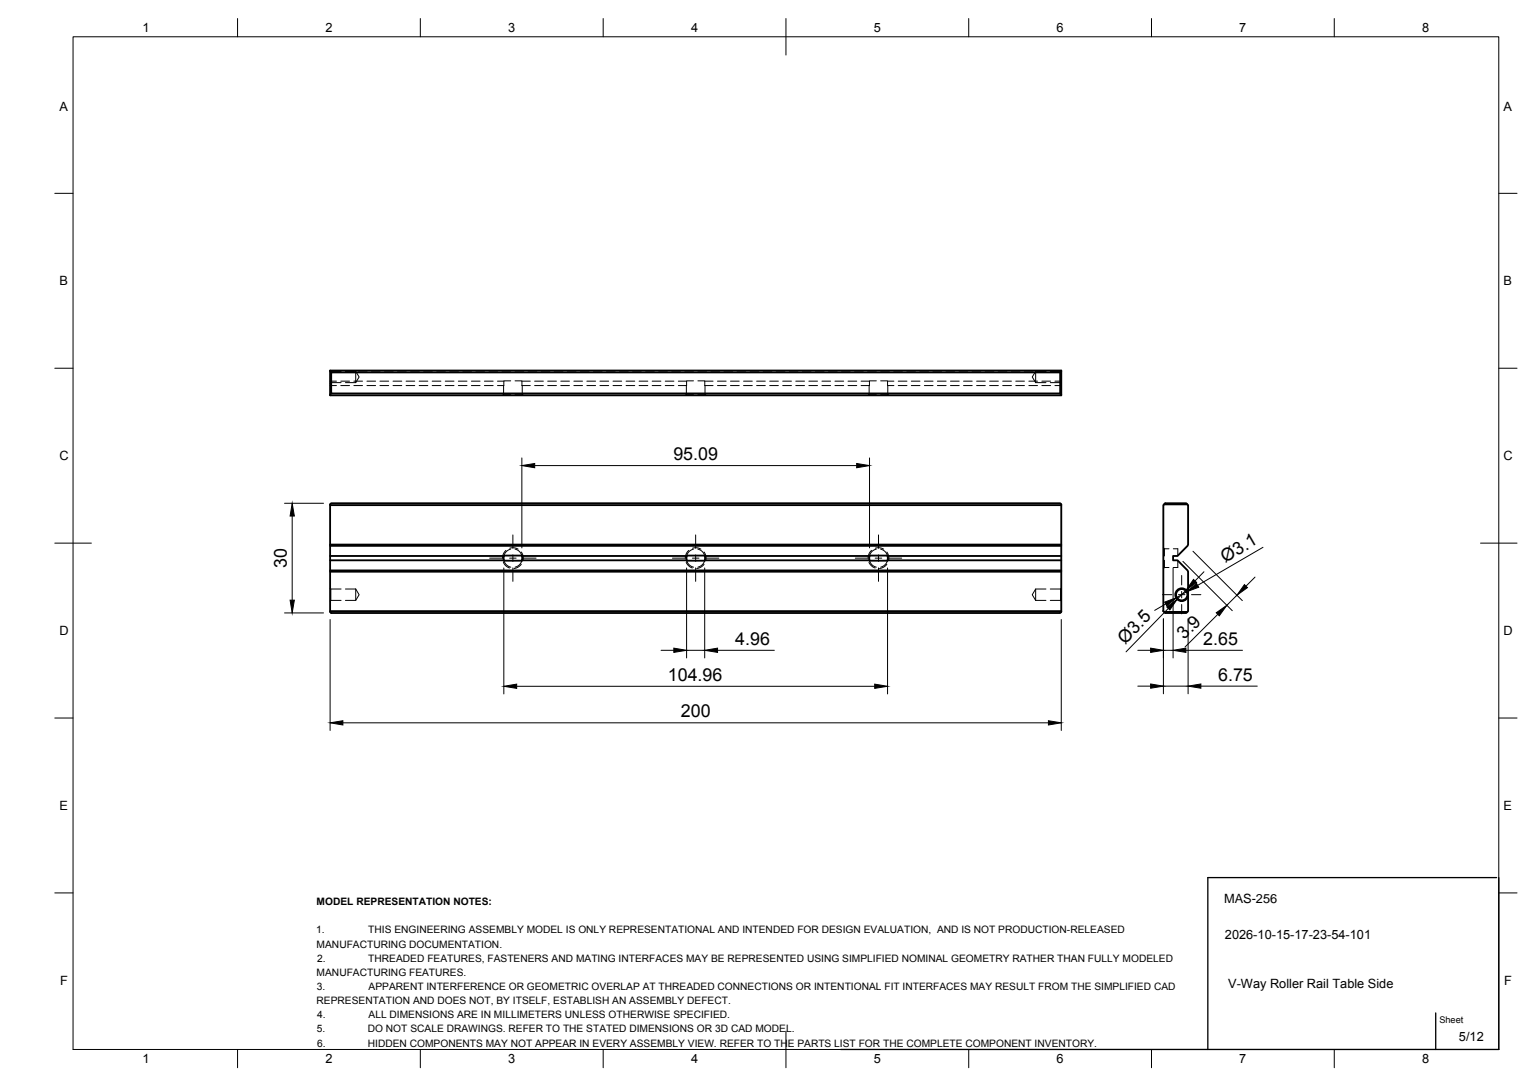
ISO-10303-21;
HEADER;
/* Generated by software containing ST-Developer
 * from STEP Tools, Inc. (www.steptools.com) 
 */

FILE_DESCRIPTION(
/* description */ (''),
/* implementation_level */ '2;1');

FILE_NAME(
/* name */ 'V-Way Roller Rail Table Side.step',
/* time_stamp */ '2026-10-14T18:40:07-07:00',
/* author */ (''),
/* organization */ (''),
/* preprocessor_version */ 'ST-DEVELOPER v20.2',
/* originating_system */ 'Autodesk Translation Framework v15.15.0.0',
/* authorisation */ '');

FILE_SCHEMA (('AUTOMOTIVE_DESIGN { 1 0 10303 214 3 1 1 }'));
ENDSEC;

DATA;
#10=MECHANICAL_DESIGN_GEOMETRIC_PRESENTATION_REPRESENTATION('',(#833),#81040);
#372=ELLIPSE('',#15639,3.6062445840514,2.55000000000001);
#373=ELLIPSE('',#15641,3.6062445840514,2.55000000000001);
#374=ELLIPSE('',#15643,3.6062445840514,2.55000000000001);
#375=ELLIPSE('',#15645,3.6062445840514,2.55000000000001);
#376=ELLIPSE('',#15651,3.6062445840514,2.55000000000001);
#377=ELLIPSE('',#15653,3.6062445840514,2.55000000000001);
#378=ELLIPSE('',#15655,3.6062445840514,2.55000000000001);
#379=ELLIPSE('',#15657,3.6062445840514,2.55000000000001);
#380=ELLIPSE('',#15663,3.60624458405139,2.55);
#381=ELLIPSE('',#15665,3.60624458405139,2.55);
#382=ELLIPSE('',#15667,3.60624458405139,2.55);
#383=ELLIPSE('',#15669,3.60624458405139,2.55);
#813=SHAPE_REPRESENTATION_RELATIONSHIP('SRR','None',#81132,#823);
#823=ADVANCED_BREP_SHAPE_REPRESENTATION('',(#843),#81032);
#833=STYLED_ITEM('',(#81191),#843);
#843=MANIFOLD_SOLID_BREP('Body1',#15086);
#915=CYLINDRICAL_SURFACE('',#15619,1.55);
#916=CYLINDRICAL_SURFACE('',#15627,1.55);
#917=CYLINDRICAL_SURFACE('',#15637,2.55000000000001);
#918=CYLINDRICAL_SURFACE('',#15649,2.55000000000001);
#919=CYLINDRICAL_SURFACE('',#15661,2.55);
#1169=FACE_BOUND('',#2653,.T.);
#1170=FACE_BOUND('',#2654,.T.);
#1171=FACE_BOUND('',#2655,.T.);
#1283=PLANE('',#15618);
#1284=PLANE('',#15626);
#1285=PLANE('',#15634);
#1286=PLANE('',#15671);
#1287=PLANE('',#15672);
#1288=PLANE('',#15673);
#1289=PLANE('',#15674);
#1290=PLANE('',#15675);
#1291=PLANE('',#15676);
#1292=PLANE('',#15677);
#1293=PLANE('',#15678);
#1294=PLANE('',#15679);
#1295=PLANE('',#15680);
#1296=PLANE('',#15681);
#1297=PLANE('',#15682);
#1298=PLANE('',#15683);
#1299=PLANE('',#15684);
#1300=PLANE('',#15685);
#1301=PLANE('',#15686);
#1302=PLANE('',#15687);
#1303=PLANE('',#15688);
#1304=PLANE('',#15689);
#1305=PLANE('',#15690);
#1306=PLANE('',#15691);
#1307=PLANE('',#15692);
#1308=PLANE('',#15693);
#1309=PLANE('',#15694);
#1310=PLANE('',#15695);
#1311=PLANE('',#15696);
#1312=PLANE('',#15697);
#1313=PLANE('',#15698);
#1314=PLANE('',#15699);
#1315=PLANE('',#15700);
#1316=PLANE('',#15701);
#1317=PLANE('',#15702);
#1318=PLANE('',#15703);
#1319=PLANE('',#15704);
#1814=FACE_OUTER_BOUND('',#2643,.T.);
#1815=FACE_OUTER_BOUND('',#2644,.T.);
#1816=FACE_OUTER_BOUND('',#2645,.T.);
#1817=FACE_OUTER_BOUND('',#2646,.T.);
#1818=FACE_OUTER_BOUND('',#2647,.T.);
#1819=FACE_OUTER_BOUND('',#2648,.T.);
#1820=FACE_OUTER_BOUND('',#2649,.T.);
#1821=FACE_OUTER_BOUND('',#2650,.T.);
#1822=FACE_OUTER_BOUND('',#2651,.T.);
#1823=FACE_OUTER_BOUND('',#2652,.T.);
#1824=FACE_OUTER_BOUND('',#2656,.T.);
#1825=FACE_OUTER_BOUND('',#2657,.T.);
#1826=FACE_OUTER_BOUND('',#2658,.T.);
#1827=FACE_OUTER_BOUND('',#2659,.T.);
#1828=FACE_OUTER_BOUND('',#2660,.T.);
#1829=FACE_OUTER_BOUND('',#2661,.T.);
#1830=FACE_OUTER_BOUND('',#2662,.T.);
#1831=FACE_OUTER_BOUND('',#2663,.T.);
#1832=FACE_OUTER_BOUND('',#2664,.T.);
#1833=FACE_OUTER_BOUND('',#2665,.T.);
#1834=FACE_OUTER_BOUND('',#2666,.T.);
#1835=FACE_OUTER_BOUND('',#2667,.T.);
#1836=FACE_OUTER_BOUND('',#2668,.T.);
#1837=FACE_OUTER_BOUND('',#2669,.T.);
#1838=FACE_OUTER_BOUND('',#2670,.T.);
#1839=FACE_OUTER_BOUND('',#2671,.T.);
#1840=FACE_OUTER_BOUND('',#2672,.T.);
#1841=FACE_OUTER_BOUND('',#2673,.T.);
#1842=FACE_OUTER_BOUND('',#2674,.T.);
#1843=FACE_OUTER_BOUND('',#2675,.T.);
#1844=FACE_OUTER_BOUND('',#2676,.T.);
#1845=FACE_OUTER_BOUND('',#2677,.T.);
#1846=FACE_OUTER_BOUND('',#2678,.T.);
#1847=FACE_OUTER_BOUND('',#2679,.T.);
#1848=FACE_OUTER_BOUND('',#2680,.T.);
#1849=FACE_OUTER_BOUND('',#2681,.T.);
#1850=FACE_OUTER_BOUND('',#2682,.T.);
#1851=FACE_OUTER_BOUND('',#2683,.T.);
#1852=FACE_OUTER_BOUND('',#2684,.T.);
#1853=FACE_OUTER_BOUND('',#2685,.T.);
#1854=FACE_OUTER_BOUND('',#2686,.T.);
#1855=FACE_OUTER_BOUND('',#2687,.T.);
#1856=FACE_OUTER_BOUND('',#2688,.T.);
#1857=FACE_OUTER_BOUND('',#2689,.T.);
#1858=FACE_OUTER_BOUND('',#2690,.T.);
#1859=FACE_OUTER_BOUND('',#2691,.T.);
#1860=FACE_OUTER_BOUND('',#2692,.T.);
#1861=FACE_OUTER_BOUND('',#2693,.T.);
#1862=FACE_OUTER_BOUND('',#2694,.T.);
#2643=EDGE_LOOP('',(#10770,#10771,#10772,#10773));
#2644=EDGE_LOOP('',(#10774,#10775,#10776,#10777,#10778,#10779,#10780,#10781,
#10782,#10783,#10784,#10785,#10786,#10787,#10788,#10789,#10790,#10791));
#2645=EDGE_LOOP('',(#10792,#10793,#10794,#10795,#10796));
#2646=EDGE_LOOP('',(#10797,#10798,#10799,#10800));
#2647=EDGE_LOOP('',(#10801,#10802,#10803,#10804));
#2648=EDGE_LOOP('',(#10805,#10806,#10807,#10808,#10809,#10810,#10811,#10812,
#10813,#10814,#10815,#10816,#10817,#10818,#10819,#10820,#10821,#10822));
#2649=EDGE_LOOP('',(#10823,#10824,#10825,#10826,#10827));
#2650=EDGE_LOOP('',(#10828,#10829,#10830,#10831));
#2651=EDGE_LOOP('',(#10832,#10833,#10834,#10835));
#2652=EDGE_LOOP('',(#10836,#10837,#10838,#10839));
#2653=EDGE_LOOP('',(#10840));
#2654=EDGE_LOOP('',(#10841));
#2655=EDGE_LOOP('',(#10842));
#2656=EDGE_LOOP('',(#10843,#10844,#10845,#10846,#10847,#10848,#10849,#10850,
#10851,#10852,#10853,#10854,#10855,#10856,#10857,#10858));
#2657=EDGE_LOOP('',(#10859,#10860,#10861,#10862));
#2658=EDGE_LOOP('',(#10863,#10864,#10865,#10866,#10867,#10868,#10869,#10870,
#10871,#10872,#10873,#10874,#10875,#10876,#10877,#10878));
#2659=EDGE_LOOP('',(#10879,#10880,#10881,#10882));
#2660=EDGE_LOOP('',(#10883,#10884,#10885,#10886,#10887,#10888,#10889,#10890,
#10891,#10892,#10893,#10894,#10895,#10896,#10897,#10898));
#2661=EDGE_LOOP('',(#10899,#10900));
#2662=EDGE_LOOP('',(#10901,#10902));
#2663=EDGE_LOOP('',(#10903,#10904));
#2664=EDGE_LOOP('',(#10905,#10906));
#2665=EDGE_LOOP('',(#10907,#10908));
#2666=EDGE_LOOP('',(#10909,#10910));
#2667=EDGE_LOOP('',(#10911,#10912,#10913,#10914,#10915,#10916,#10917,#10918,
#10919,#10920,#10921,#10922,#10923,#10924,#10925,#10926));
#2668=EDGE_LOOP('',(#10927,#10928,#10929,#10930));
#2669=EDGE_LOOP('',(#10931,#10932,#10933,#10934));
#2670=EDGE_LOOP('',(#10935,#10936,#10937,#10938));
#2671=EDGE_LOOP('',(#10939,#10940,#10941,#10942));
#2672=EDGE_LOOP('',(#10943,#10944,#10945,#10946,#10947));
#2673=EDGE_LOOP('',(#10948,#10949,#10950,#10951,#10952));
#2674=EDGE_LOOP('',(#10953,#10954,#10955,#10956));
#2675=EDGE_LOOP('',(#10957,#10958,#10959,#10960));
#2676=EDGE_LOOP('',(#10961,#10962,#10963,#10964));
#2677=EDGE_LOOP('',(#10965,#10966,#10967,#10968));
#2678=EDGE_LOOP('',(#10969,#10970,#10971,#10972));
#2679=EDGE_LOOP('',(#10973,#10974,#10975,#10976,#10977,#10978));
#2680=EDGE_LOOP('',(#10979,#10980,#10981,#10982));
#2681=EDGE_LOOP('',(#10983,#10984,#10985,#10986,#10987,#10988));
#2682=EDGE_LOOP('',(#10989,#10990,#10991,#10992));
#2683=EDGE_LOOP('',(#10993,#10994,#10995,#10996));
#2684=EDGE_LOOP('',(#10997,#10998,#10999,#11000));
#2685=EDGE_LOOP('',(#11001,#11002,#11003,#11004));
#2686=EDGE_LOOP('',(#11005,#11006,#11007,#11008));
#2687=EDGE_LOOP('',(#11009,#11010,#11011,#11012));
#2688=EDGE_LOOP('',(#11013,#11014,#11015,#11016,#11017,#11018,#11019,#11020,
#11021,#11022,#11023,#11024,#11025,#11026,#11027,#11028));
#2689=EDGE_LOOP('',(#11029,#11030,#11031,#11032,#11033,#11034));
#2690=EDGE_LOOP('',(#11035,#11036,#11037,#11038,#11039,#11040));
#2691=EDGE_LOOP('',(#11041,#11042,#11043,#11044,#11045,#11046));
#2692=EDGE_LOOP('',(#11047,#11048,#11049,#11050));
#2693=EDGE_LOOP('',(#11051,#11052,#11053,#11054,#11055));
#2694=EDGE_LOOP('',(#11056,#11057,#11058,#11059));
#3510=LINE('',#21622,#4622);
#3511=LINE('',#21627,#4623);
#3512=LINE('',#21629,#4624);
#3513=LINE('',#21631,#4625);
#3514=LINE('',#21633,#4626);
#3515=LINE('',#21635,#4627);
#3516=LINE('',#21637,#4628);
#3517=LINE('',#21639,#4629);
#3518=LINE('',#21641,#4630);
#3519=LINE('',#21643,#4631);
#3520=LINE('',#21645,#4632);
#3521=LINE('',#21647,#4633);
#3522=LINE('',#21649,#4634);
#3523=LINE('',#21651,#4635);
#3524=LINE('',#21653,#4636);
#3525=LINE('',#21654,#4637);
#3526=LINE('',#21656,#4638);
#3527=LINE('',#21657,#4639);
#3528=LINE('',#21660,#4640);
#3529=LINE('',#21666,#4641);
#3530=LINE('',#21671,#4642);
#3531=LINE('',#21676,#4643);
#3532=LINE('',#21678,#4644);
#3533=LINE('',#21679,#4645);
#3534=LINE('',#21681,#4646);
#3535=LINE('',#21683,#4647);
#3536=LINE('',#21685,#4648);
#3537=LINE('',#21687,#4649);
#3538=LINE('',#21689,#4650);
#3539=LINE('',#21691,#4651);
#3540=LINE('',#21693,#4652);
#3541=LINE('',#21695,#4653);
#3542=LINE('',#21697,#4654);
#3543=LINE('',#21699,#4655);
#3544=LINE('',#21701,#4656);
#3545=LINE('',#21703,#4657);
#3546=LINE('',#21705,#4658);
#3547=LINE('',#21706,#4659);
#3548=LINE('',#21709,#4660);
#3549=LINE('',#21715,#4661);
#3550=LINE('',#21720,#4662);
#3551=LINE('',#21723,#4663);
#3552=LINE('',#21724,#4664);
#3553=LINE('',#21731,#4665);
#3554=LINE('',#21735,#4666);
#3555=LINE('',#21743,#4667);
#3556=LINE('',#21747,#4668);
#3557=LINE('',#21755,#4669);
#3558=LINE('',#21760,#4670);
#3559=LINE('',#21763,#4671);
#3560=LINE('',#21767,#4672);
#3561=LINE('',#21775,#4673);
#3562=LINE('',#21779,#4674);
#3563=LINE('',#21787,#4675);
#3564=LINE('',#21792,#4676);
#3565=LINE('',#21795,#4677);
#3566=LINE('',#21799,#4678);
#3567=LINE('',#21807,#4679);
#3568=LINE('',#21811,#4680);
#3569=LINE('',#21819,#4681);
#3570=LINE('',#21822,#4682);
#3571=LINE('',#21824,#4683);
#3572=LINE('',#21826,#4684);
#3573=LINE('',#21828,#4685);
#3574=LINE('',#21830,#4686);
#3575=LINE('',#21832,#4687);
#3576=LINE('',#21834,#4688);
#3577=LINE('',#21835,#4689);
#3578=LINE('',#21836,#4690);
#3579=LINE('',#21837,#4691);
#3580=LINE('',#21838,#4692);
#3581=LINE('',#21840,#4693);
#3582=LINE('',#21842,#4694);
#3583=LINE('',#21844,#4695);
#3584=LINE('',#21846,#4696);
#3585=LINE('',#21848,#4697);
#3586=LINE('',#21850,#4698);
#3587=LINE('',#21852,#4699);
#3588=LINE('',#21854,#4700);
#3589=LINE('',#21856,#4701);
#3590=LINE('',#21859,#4702);
#3591=LINE('',#21861,#4703);
#3592=LINE('',#21862,#4704);
#3593=LINE('',#21865,#4705);
#3594=LINE('',#21867,#4706);
#3595=LINE('',#21868,#4707);
#3596=LINE('',#21870,#4708);
#3597=LINE('',#21871,#4709);
#3598=LINE('',#21874,#4710);
#3599=LINE('',#21876,#4711);
#3600=LINE('',#21877,#4712);
#3601=LINE('',#21880,#4713);
#3602=LINE('',#21881,#4714);
#3603=LINE('',#21882,#4715);
#3604=LINE('',#21885,#4716);
#3605=LINE('',#21886,#4717);
#3606=LINE('',#21888,#4718);
#3607=LINE('',#21890,#4719);
#3608=LINE('',#21892,#4720);
#3609=LINE('',#21895,#4721);
#3610=LINE('',#21896,#4722);
#3611=LINE('',#21898,#4723);
#3612=LINE('',#21903,#4724);
#3613=LINE('',#21905,#4725);
#4622=VECTOR('',#17734,1.65);
#4623=VECTOR('',#17739,10.);
#4624=VECTOR('',#17740,10.);
#4625=VECTOR('',#17741,10.);
#4626=VECTOR('',#17742,10.);
#4627=VECTOR('',#17743,10.);
#4628=VECTOR('',#17744,10.);
#4629=VECTOR('',#17745,10.);
#4630=VECTOR('',#17746,10.);
#4631=VECTOR('',#17747,9.99999999999999);
#4632=VECTOR('',#17748,10.);
#4633=VECTOR('',#17749,10.);
#4634=VECTOR('',#17750,10.);
#4635=VECTOR('',#17751,10.);
#4636=VECTOR('',#17752,9.99999999999999);
#4637=VECTOR('',#17753,10.);
#4638=VECTOR('',#17754,10.);
#4639=VECTOR('',#17755,10.);
#4640=VECTOR('',#17758,1.55);
#4641=VECTOR('',#17765,0.775000000000001);
#4642=VECTOR('',#17770,1.65);
#4643=VECTOR('',#17775,10.);
#4644=VECTOR('',#17776,10.);
#4645=VECTOR('',#17777,10.);
#4646=VECTOR('',#17778,10.);
#4647=VECTOR('',#17779,9.99999999999999);
#4648=VECTOR('',#17780,10.);
#4649=VECTOR('',#17781,10.);
#4650=VECTOR('',#17782,10.);
#4651=VECTOR('',#17783,10.);
#4652=VECTOR('',#17784,9.99999999999999);
#4653=VECTOR('',#17785,10.);
#4654=VECTOR('',#17786,10.);
#4655=VECTOR('',#17787,10.);
#4656=VECTOR('',#17788,10.);
#4657=VECTOR('',#17789,10.);
#4658=VECTOR('',#17790,10.);
#4659=VECTOR('',#17791,10.);
#4660=VECTOR('',#17794,1.55);
#4661=VECTOR('',#17801,1.55);
#4662=VECTOR('',#17806,2.7);
#4663=VECTOR('',#17811,10.);
#4664=VECTOR('',#17812,10.);
#4665=VECTOR('',#17819,2.55000000000001);
#4666=VECTOR('',#17822,10.);
#4667=VECTOR('',#17829,10.);
#4668=VECTOR('',#17832,10.);
#4669=VECTOR('',#17839,10.);
#4670=VECTOR('',#17846,2.7);
#4671=VECTOR('',#17849,2.55000000000001);
#4672=VECTOR('',#17852,10.);
#4673=VECTOR('',#17859,10.);
#4674=VECTOR('',#17862,10.);
#4675=VECTOR('',#17869,10.);
#4676=VECTOR('',#17876,2.7);
#4677=VECTOR('',#17879,2.55);
#4678=VECTOR('',#17882,10.);
#4679=VECTOR('',#17889,10.);
#4680=VECTOR('',#17892,10.);
#4681=VECTOR('',#17899,10.);
#4682=VECTOR('',#17904,10.);
#4683=VECTOR('',#17907,10.);
#4684=VECTOR('',#17910,10.);
#4685=VECTOR('',#17913,10.);
#4686=VECTOR('',#17916,10.);
#4687=VECTOR('',#17919,10.);
#4688=VECTOR('',#17922,10.);
#4689=VECTOR('',#17923,10.);
#4690=VECTOR('',#17924,10.);
#4691=VECTOR('',#17925,10.);
#4692=VECTOR('',#17926,10.);
#4693=VECTOR('',#17929,10.);
#4694=VECTOR('',#17932,10.);
#4695=VECTOR('',#17935,10.);
#4696=VECTOR('',#17938,10.);
#4697=VECTOR('',#17941,10.);
#4698=VECTOR('',#17944,10.);
#4699=VECTOR('',#17947,10.);
#4700=VECTOR('',#17950,10.);
#4701=VECTOR('',#17953,10.);
#4702=VECTOR('',#17956,10.);
#4703=VECTOR('',#17957,10.);
#4704=VECTOR('',#17958,10.);
#4705=VECTOR('',#17961,10.);
#4706=VECTOR('',#17962,10.);
#4707=VECTOR('',#17963,10.);
#4708=VECTOR('',#17966,10.);
#4709=VECTOR('',#17967,10.);
#4710=VECTOR('',#17970,10.);
#4711=VECTOR('',#17971,10.);
#4712=VECTOR('',#17972,10.);
#4713=VECTOR('',#17975,10.);
#4714=VECTOR('',#17976,10.);
#4715=VECTOR('',#17977,10.);
#4716=VECTOR('',#17980,10.);
#4717=VECTOR('',#17981,10.);
#4718=VECTOR('',#17984,10.);
#4719=VECTOR('',#17987,10.);
#4720=VECTOR('',#17990,10.);
#4721=VECTOR('',#17995,10.);
#4722=VECTOR('',#17996,10.);
#4723=VECTOR('',#17999,10.);
#4724=VECTOR('',#18008,10.);
#4725=VECTOR('',#18011,10.);
#5642=CIRCLE('',#15616,1.55);
#5643=CIRCLE('',#15617,1.75);
#5644=CIRCLE('',#15620,1.55);
#5645=CIRCLE('',#15621,1.55);
#5646=CIRCLE('',#15624,1.55);
#5647=CIRCLE('',#15625,1.75);
#5648=CIRCLE('',#15628,1.55);
#5649=CIRCLE('',#15629,1.55);
#5650=CIRCLE('',#15632,2.55000000000001);
#5651=CIRCLE('',#15633,2.85);
#5652=CIRCLE('',#15635,2.85);
#5653=CIRCLE('',#15636,2.85);
#5654=CIRCLE('',#15638,2.55000000000001);
#5655=CIRCLE('',#15640,2.55000000000001);
#5656=CIRCLE('',#15642,2.55000000000001);
#5657=CIRCLE('',#15644,2.55000000000001);
#5658=CIRCLE('',#15646,2.55000000000001);
#5659=CIRCLE('',#15648,2.55000000000001);
#5660=CIRCLE('',#15650,2.55000000000001);
#5661=CIRCLE('',#15652,2.55000000000001);
#5662=CIRCLE('',#15654,2.55000000000001);
#5663=CIRCLE('',#15656,2.55000000000001);
#5664=CIRCLE('',#15658,2.55000000000001);
#5665=CIRCLE('',#15660,2.55);
#5666=CIRCLE('',#15662,2.55);
#5667=CIRCLE('',#15664,2.55);
#5668=CIRCLE('',#15666,2.55);
#5669=CIRCLE('',#15668,2.55);
#5670=CIRCLE('',#15670,2.55);
#6341=VERTEX_POINT('',#21619);
#6342=VERTEX_POINT('',#21621);
#6343=VERTEX_POINT('',#21625);
#6344=VERTEX_POINT('',#21626);
#6345=VERTEX_POINT('',#21628);
#6346=VERTEX_POINT('',#21630);
#6347=VERTEX_POINT('',#21632);
#6348=VERTEX_POINT('',#21634);
#6349=VERTEX_POINT('',#21636);
#6350=VERTEX_POINT('',#21638);
#6351=VERTEX_POINT('',#21640);
#6352=VERTEX_POINT('',#21642);
#6353=VERTEX_POINT('',#21644);
#6354=VERTEX_POINT('',#21646);
#6355=VERTEX_POINT('',#21648);
#6356=VERTEX_POINT('',#21650);
#6357=VERTEX_POINT('',#21652);
#6358=VERTEX_POINT('',#21655);
#6359=VERTEX_POINT('',#21659);
#6360=VERTEX_POINT('',#21661);
#6361=VERTEX_POINT('',#21665);
#6362=VERTEX_POINT('',#21668);
#6363=VERTEX_POINT('',#21670);
#6364=VERTEX_POINT('',#21674);
#6365=VERTEX_POINT('',#21675);
#6366=VERTEX_POINT('',#21677);
#6367=VERTEX_POINT('',#21680);
#6368=VERTEX_POINT('',#21682);
#6369=VERTEX_POINT('',#21684);
#6370=VERTEX_POINT('',#21686);
#6371=VERTEX_POINT('',#21688);
#6372=VERTEX_POINT('',#21690);
#6373=VERTEX_POINT('',#21692);
#6374=VERTEX_POINT('',#21694);
#6375=VERTEX_POINT('',#21696);
#6376=VERTEX_POINT('',#21698);
#6377=VERTEX_POINT('',#21700);
#6378=VERTEX_POINT('',#21702);
#6379=VERTEX_POINT('',#21704);
#6380=VERTEX_POINT('',#21708);
#6381=VERTEX_POINT('',#21710);
#6382=VERTEX_POINT('',#21714);
#6383=VERTEX_POINT('',#21717);
#6384=VERTEX_POINT('',#21719);
#6385=VERTEX_POINT('',#21725);
#6386=VERTEX_POINT('',#21727);
#6387=VERTEX_POINT('',#21730);
#6388=VERTEX_POINT('',#21732);
#6389=VERTEX_POINT('',#21734);
#6390=VERTEX_POINT('',#21736);
#6391=VERTEX_POINT('',#21738);
#6392=VERTEX_POINT('',#21740);
#6393=VERTEX_POINT('',#21742);
#6394=VERTEX_POINT('',#21744);
#6395=VERTEX_POINT('',#21746);
#6396=VERTEX_POINT('',#21748);
#6397=VERTEX_POINT('',#21750);
#6398=VERTEX_POINT('',#21752);
#6399=VERTEX_POINT('',#21754);
#6400=VERTEX_POINT('',#21758);
#6401=VERTEX_POINT('',#21762);
#6402=VERTEX_POINT('',#21764);
#6403=VERTEX_POINT('',#21766);
#6404=VERTEX_POINT('',#21768);
#6405=VERTEX_POINT('',#21770);
#6406=VERTEX_POINT('',#21772);
#6407=VERTEX_POINT('',#21774);
#6408=VERTEX_POINT('',#21776);
#6409=VERTEX_POINT('',#21778);
#6410=VERTEX_POINT('',#21780);
#6411=VERTEX_POINT('',#21782);
#6412=VERTEX_POINT('',#21784);
#6413=VERTEX_POINT('',#21786);
#6414=VERTEX_POINT('',#21790);
#6415=VERTEX_POINT('',#21794);
#6416=VERTEX_POINT('',#21796);
#6417=VERTEX_POINT('',#21798);
#6418=VERTEX_POINT('',#21800);
#6419=VERTEX_POINT('',#21802);
#6420=VERTEX_POINT('',#21804);
#6421=VERTEX_POINT('',#21806);
#6422=VERTEX_POINT('',#21808);
#6423=VERTEX_POINT('',#21810);
#6424=VERTEX_POINT('',#21812);
#6425=VERTEX_POINT('',#21814);
#6426=VERTEX_POINT('',#21816);
#6427=VERTEX_POINT('',#21818);
#6428=VERTEX_POINT('',#21858);
#6429=VERTEX_POINT('',#21860);
#6430=VERTEX_POINT('',#21864);
#6431=VERTEX_POINT('',#21866);
#6432=VERTEX_POINT('',#21873);
#6433=VERTEX_POINT('',#21875);
#6434=VERTEX_POINT('',#21879);
#6435=VERTEX_POINT('',#21884);
#8048=EDGE_CURVE('',#6341,#6341,#5642,.T.);
#8049=EDGE_CURVE('',#6341,#6342,#3510,.T.);
#8050=EDGE_CURVE('',#6342,#6342,#5643,.T.);
#8051=EDGE_CURVE('',#6343,#6344,#3511,.T.);
#8052=EDGE_CURVE('',#6345,#6343,#3512,.T.);
#8053=EDGE_CURVE('',#6345,#6346,#3513,.T.);
#8054=EDGE_CURVE('',#6347,#6346,#3514,.T.);
#8055=EDGE_CURVE('',#6348,#6347,#3515,.T.);
#8056=EDGE_CURVE('',#6349,#6348,#3516,.T.);
#8057=EDGE_CURVE('',#6349,#6350,#3517,.T.);
#8058=EDGE_CURVE('',#6351,#6350,#3518,.T.);
#8059=EDGE_CURVE('',#6351,#6352,#3519,.T.);
#8060=EDGE_CURVE('',#6352,#6353,#3520,.T.);
#8061=EDGE_CURVE('',#6353,#6354,#3521,.T.);
#8062=EDGE_CURVE('',#6354,#6355,#3522,.T.);
#8063=EDGE_CURVE('',#6355,#6356,#3523,.T.);
#8064=EDGE_CURVE('',#6357,#6356,#3524,.T.);
#8065=EDGE_CURVE('',#6357,#6342,#3525,.T.);
#8066=EDGE_CURVE('',#6342,#6358,#3526,.T.);
#8067=EDGE_CURVE('',#6344,#6358,#3527,.T.);
#8068=EDGE_CURVE('',#6341,#6359,#3528,.T.);
#8069=EDGE_CURVE('',#6359,#6360,#5644,.T.);
#8070=EDGE_CURVE('',#6360,#6359,#5645,.T.);
#8071=EDGE_CURVE('',#6361,#6360,#3529,.T.);
#8072=EDGE_CURVE('',#6362,#6362,#5646,.T.);
#8073=EDGE_CURVE('',#6362,#6363,#3530,.T.);
#8074=EDGE_CURVE('',#6363,#6363,#5647,.T.);
#8075=EDGE_CURVE('',#6364,#6365,#3531,.T.);
#8076=EDGE_CURVE('',#6366,#6364,#3532,.T.);
#8077=EDGE_CURVE('',#6366,#6363,#3533,.T.);
#8078=EDGE_CURVE('',#6363,#6367,#3534,.T.);
#8079=EDGE_CURVE('',#6368,#6367,#3535,.T.);
#8080=EDGE_CURVE('',#6368,#6369,#3536,.T.);
#8081=EDGE_CURVE('',#6369,#6370,#3537,.T.);
#8082=EDGE_CURVE('',#6370,#6371,#3538,.T.);
#8083=EDGE_CURVE('',#6371,#6372,#3539,.T.);
#8084=EDGE_CURVE('',#6372,#6373,#3540,.T.);
#8085=EDGE_CURVE('',#6374,#6373,#3541,.T.);
#8086=EDGE_CURVE('',#6374,#6375,#3542,.T.);
#8087=EDGE_CURVE('',#6376,#6375,#3543,.T.);
#8088=EDGE_CURVE('',#6377,#6376,#3544,.T.);
#8089=EDGE_CURVE('',#6378,#6377,#3545,.T.);
#8090=EDGE_CURVE('',#6378,#6379,#3546,.T.);
#8091=EDGE_CURVE('',#6365,#6379,#3547,.T.);
#8092=EDGE_CURVE('',#6362,#6380,#3548,.T.);
#8093=EDGE_CURVE('',#6380,#6381,#5648,.T.);
#8094=EDGE_CURVE('',#6381,#6380,#5649,.T.);
#8095=EDGE_CURVE('',#6382,#6381,#3549,.T.);
#8096=EDGE_CURVE('',#6383,#6383,#5650,.T.);
#8097=EDGE_CURVE('',#6383,#6384,#3550,.T.);
#8098=EDGE_CURVE('',#6384,#6384,#5651,.T.);
#8099=EDGE_CURVE('',#6379,#6345,#3551,.T.);
#8100=EDGE_CURVE('',#6346,#6378,#3552,.T.);
#8101=EDGE_CURVE('',#6385,#6385,#5652,.T.);
#8102=EDGE_CURVE('',#6386,#6386,#5653,.T.);
#8103=EDGE_CURVE('',#6383,#6387,#3553,.T.);
#8104=EDGE_CURVE('',#6388,#6387,#5654,.T.);
#8105=EDGE_CURVE('',#6389,#6388,#3554,.T.);
#8106=EDGE_CURVE('',#6390,#6389,#372,.T.);
#8107=EDGE_CURVE('',#6390,#6391,#5655,.T.);
#8108=EDGE_CURVE('',#6392,#6391,#373,.T.);
#8109=EDGE_CURVE('',#6393,#6392,#3555,.T.);
#8110=EDGE_CURVE('',#6394,#6393,#5656,.T.);
#8111=EDGE_CURVE('',#6395,#6394,#3556,.T.);
#8112=EDGE_CURVE('',#6396,#6395,#374,.T.);
#8113=EDGE_CURVE('',#6396,#6397,#5657,.T.);
#8114=EDGE_CURVE('',#6398,#6397,#375,.T.);
#8115=EDGE_CURVE('',#6399,#6398,#3557,.T.);
#8116=EDGE_CURVE('',#6387,#6399,#5658,.T.);
#8117=EDGE_CURVE('',#6400,#6400,#5659,.T.);
#8118=EDGE_CURVE('',#6400,#6385,#3558,.T.);
#8119=EDGE_CURVE('',#6400,#6401,#3559,.T.);
#8120=EDGE_CURVE('',#6402,#6401,#5660,.T.);
#8121=EDGE_CURVE('',#6403,#6402,#3560,.T.);
#8122=EDGE_CURVE('',#6404,#6403,#376,.T.);
#8123=EDGE_CURVE('',#6404,#6405,#5661,.T.);
#8124=EDGE_CURVE('',#6406,#6405,#377,.T.);
#8125=EDGE_CURVE('',#6407,#6406,#3561,.T.);
#8126=EDGE_CURVE('',#6408,#6407,#5662,.T.);
#8127=EDGE_CURVE('',#6409,#6408,#3562,.T.);
#8128=EDGE_CURVE('',#6410,#6409,#378,.T.);
#8129=EDGE_CURVE('',#6410,#6411,#5663,.T.);
#8130=EDGE_CURVE('',#6412,#6411,#379,.T.);
#8131=EDGE_CURVE('',#6413,#6412,#3563,.T.);
#8132=EDGE_CURVE('',#6401,#6413,#5664,.T.);
#8133=EDGE_CURVE('',#6414,#6414,#5665,.T.);
#8134=EDGE_CURVE('',#6414,#6386,#3564,.T.);
#8135=EDGE_CURVE('',#6414,#6415,#3565,.T.);
#8136=EDGE_CURVE('',#6416,#6415,#5666,.T.);
#8137=EDGE_CURVE('',#6417,#6416,#3566,.T.);
#8138=EDGE_CURVE('',#6418,#6417,#380,.T.);
#8139=EDGE_CURVE('',#6418,#6419,#5667,.T.);
#8140=EDGE_CURVE('',#6420,#6419,#381,.T.);
#8141=EDGE_CURVE('',#6421,#6420,#3567,.T.);
#8142=EDGE_CURVE('',#6422,#6421,#5668,.T.);
#8143=EDGE_CURVE('',#6423,#6422,#3568,.T.);
#8144=EDGE_CURVE('',#6424,#6423,#382,.T.);
#8145=EDGE_CURVE('',#6424,#6425,#5669,.T.);
#8146=EDGE_CURVE('',#6426,#6425,#383,.T.);
#8147=EDGE_CURVE('',#6427,#6426,#3569,.T.);
#8148=EDGE_CURVE('',#6415,#6427,#5670,.T.);
#8149=EDGE_CURVE('',#6419,#6418,#3570,.T.);
#8150=EDGE_CURVE('',#6425,#6424,#3571,.T.);
#8151=EDGE_CURVE('',#6405,#6404,#3572,.T.);
#8152=EDGE_CURVE('',#6411,#6410,#3573,.T.);
#8153=EDGE_CURVE('',#6391,#6390,#3574,.T.);
#8154=EDGE_CURVE('',#6397,#6396,#3575,.T.);
#8155=EDGE_CURVE('',#6423,#6412,#3576,.T.);
#8156=EDGE_CURVE('',#6409,#6398,#3577,.T.);
#8157=EDGE_CURVE('',#6395,#6352,#3578,.T.);
#8158=EDGE_CURVE('',#6373,#6351,#3579,.T.);
#8159=EDGE_CURVE('',#6372,#6426,#3580,.T.);
#8160=EDGE_CURVE('',#6394,#6353,#3581,.T.);
#8161=EDGE_CURVE('',#6408,#6399,#3582,.T.);
#8162=EDGE_CURVE('',#6422,#6413,#3583,.T.);
#8163=EDGE_CURVE('',#6393,#6354,#3584,.T.);
#8164=EDGE_CURVE('',#6407,#6388,#3585,.T.);
#8165=EDGE_CURVE('',#6421,#6402,#3586,.T.);
#8166=EDGE_CURVE('',#6392,#6355,#3587,.T.);
#8167=EDGE_CURVE('',#6406,#6389,#3588,.T.);
#8168=EDGE_CURVE('',#6420,#6403,#3589,.T.);
#8169=EDGE_CURVE('',#6428,#6343,#3590,.T.);
#8170=EDGE_CURVE('',#6344,#6429,#3591,.T.);
#8171=EDGE_CURVE('',#6429,#6428,#3592,.T.);
#8172=EDGE_CURVE('',#6430,#6429,#3593,.T.);
#8173=EDGE_CURVE('',#6431,#6430,#3594,.T.);
#8174=EDGE_CURVE('',#6428,#6431,#3595,.T.);
#8175=EDGE_CURVE('',#6358,#6366,#3596,.T.);
#8176=EDGE_CURVE('',#6430,#6364,#3597,.T.);
#8177=EDGE_CURVE('',#6432,#6348,#3598,.T.);
#8178=EDGE_CURVE('',#6347,#6433,#3599,.T.);
#8179=EDGE_CURVE('',#6433,#6432,#3600,.T.);
#8180=EDGE_CURVE('',#6432,#6434,#3601,.T.);
#8181=EDGE_CURVE('',#6376,#6434,#3602,.T.);
#8182=EDGE_CURVE('',#6375,#6349,#3603,.T.);
#8183=EDGE_CURVE('',#6435,#6433,#3604,.T.);
#8184=EDGE_CURVE('',#6434,#6435,#3605,.T.);
#8185=EDGE_CURVE('',#6365,#6431,#3606,.T.);
#8186=EDGE_CURVE('',#6435,#6377,#3607,.T.);
#8187=EDGE_CURVE('',#6350,#6374,#3608,.T.);
#8188=EDGE_CURVE('',#6356,#6368,#3609,.T.);
#8189=EDGE_CURVE('',#6367,#6357,#3610,.T.);
#8190=EDGE_CURVE('',#6369,#6417,#3611,.T.);
#8191=EDGE_CURVE('',#6370,#6416,#3612,.T.);
#8192=EDGE_CURVE('',#6371,#6427,#3613,.T.);
#10770=ORIENTED_EDGE('',*,*,#8048,.T.);
#10771=ORIENTED_EDGE('',*,*,#8049,.T.);
#10772=ORIENTED_EDGE('',*,*,#8050,.T.);
#10773=ORIENTED_EDGE('',*,*,#8049,.F.);
#10774=ORIENTED_EDGE('',*,*,#8051,.F.);
#10775=ORIENTED_EDGE('',*,*,#8052,.F.);
#10776=ORIENTED_EDGE('',*,*,#8053,.T.);
#10777=ORIENTED_EDGE('',*,*,#8054,.F.);
#10778=ORIENTED_EDGE('',*,*,#8055,.F.);
#10779=ORIENTED_EDGE('',*,*,#8056,.F.);
#10780=ORIENTED_EDGE('',*,*,#8057,.T.);
#10781=ORIENTED_EDGE('',*,*,#8058,.F.);
#10782=ORIENTED_EDGE('',*,*,#8059,.T.);
#10783=ORIENTED_EDGE('',*,*,#8060,.T.);
#10784=ORIENTED_EDGE('',*,*,#8061,.T.);
#10785=ORIENTED_EDGE('',*,*,#8062,.T.);
#10786=ORIENTED_EDGE('',*,*,#8063,.T.);
#10787=ORIENTED_EDGE('',*,*,#8064,.F.);
#10788=ORIENTED_EDGE('',*,*,#8065,.T.);
#10789=ORIENTED_EDGE('',*,*,#8050,.F.);
#10790=ORIENTED_EDGE('',*,*,#8066,.T.);
#10791=ORIENTED_EDGE('',*,*,#8067,.F.);
#10792=ORIENTED_EDGE('',*,*,#8048,.F.);
#10793=ORIENTED_EDGE('',*,*,#8068,.T.);
#10794=ORIENTED_EDGE('',*,*,#8069,.T.);
#10795=ORIENTED_EDGE('',*,*,#8070,.T.);
#10796=ORIENTED_EDGE('',*,*,#8068,.F.);
#10797=ORIENTED_EDGE('',*,*,#8071,.T.);
#10798=ORIENTED_EDGE('',*,*,#8069,.F.);
#10799=ORIENTED_EDGE('',*,*,#8070,.F.);
#10800=ORIENTED_EDGE('',*,*,#8071,.F.);
#10801=ORIENTED_EDGE('',*,*,#8072,.T.);
#10802=ORIENTED_EDGE('',*,*,#8073,.T.);
#10803=ORIENTED_EDGE('',*,*,#8074,.T.);
#10804=ORIENTED_EDGE('',*,*,#8073,.F.);
#10805=ORIENTED_EDGE('',*,*,#8075,.F.);
#10806=ORIENTED_EDGE('',*,*,#8076,.F.);
#10807=ORIENTED_EDGE('',*,*,#8077,.T.);
#10808=ORIENTED_EDGE('',*,*,#8074,.F.);
#10809=ORIENTED_EDGE('',*,*,#8078,.T.);
#10810=ORIENTED_EDGE('',*,*,#8079,.F.);
#10811=ORIENTED_EDGE('',*,*,#8080,.T.);
#10812=ORIENTED_EDGE('',*,*,#8081,.T.);
#10813=ORIENTED_EDGE('',*,*,#8082,.T.);
#10814=ORIENTED_EDGE('',*,*,#8083,.T.);
#10815=ORIENTED_EDGE('',*,*,#8084,.T.);
#10816=ORIENTED_EDGE('',*,*,#8085,.F.);
#10817=ORIENTED_EDGE('',*,*,#8086,.T.);
#10818=ORIENTED_EDGE('',*,*,#8087,.F.);
#10819=ORIENTED_EDGE('',*,*,#8088,.F.);
#10820=ORIENTED_EDGE('',*,*,#8089,.F.);
#10821=ORIENTED_EDGE('',*,*,#8090,.T.);
#10822=ORIENTED_EDGE('',*,*,#8091,.F.);
#10823=ORIENTED_EDGE('',*,*,#8072,.F.);
#10824=ORIENTED_EDGE('',*,*,#8092,.T.);
#10825=ORIENTED_EDGE('',*,*,#8093,.T.);
#10826=ORIENTED_EDGE('',*,*,#8094,.T.);
#10827=ORIENTED_EDGE('',*,*,#8092,.F.);
#10828=ORIENTED_EDGE('',*,*,#8095,.T.);
#10829=ORIENTED_EDGE('',*,*,#8093,.F.);
#10830=ORIENTED_EDGE('',*,*,#8094,.F.);
#10831=ORIENTED_EDGE('',*,*,#8095,.F.);
#10832=ORIENTED_EDGE('',*,*,#8096,.T.);
#10833=ORIENTED_EDGE('',*,*,#8097,.T.);
#10834=ORIENTED_EDGE('',*,*,#8098,.T.);
#10835=ORIENTED_EDGE('',*,*,#8097,.F.);
#10836=ORIENTED_EDGE('',*,*,#8099,.F.);
#10837=ORIENTED_EDGE('',*,*,#8090,.F.);
#10838=ORIENTED_EDGE('',*,*,#8100,.F.);
#10839=ORIENTED_EDGE('',*,*,#8053,.F.);
#10840=ORIENTED_EDGE('',*,*,#8101,.F.);
#10841=ORIENTED_EDGE('',*,*,#8102,.F.);
#10842=ORIENTED_EDGE('',*,*,#8098,.F.);
#10843=ORIENTED_EDGE('',*,*,#8096,.F.);
#10844=ORIENTED_EDGE('',*,*,#8103,.T.);
#10845=ORIENTED_EDGE('',*,*,#8104,.F.);
#10846=ORIENTED_EDGE('',*,*,#8105,.F.);
#10847=ORIENTED_EDGE('',*,*,#8106,.F.);
#10848=ORIENTED_EDGE('',*,*,#8107,.T.);
#10849=ORIENTED_EDGE('',*,*,#8108,.F.);
#10850=ORIENTED_EDGE('',*,*,#8109,.F.);
#10851=ORIENTED_EDGE('',*,*,#8110,.F.);
#10852=ORIENTED_EDGE('',*,*,#8111,.F.);
#10853=ORIENTED_EDGE('',*,*,#8112,.F.);
#10854=ORIENTED_EDGE('',*,*,#8113,.T.);
#10855=ORIENTED_EDGE('',*,*,#8114,.F.);
#10856=ORIENTED_EDGE('',*,*,#8115,.F.);
#10857=ORIENTED_EDGE('',*,*,#8116,.F.);
#10858=ORIENTED_EDGE('',*,*,#8103,.F.);
#10859=ORIENTED_EDGE('',*,*,#8117,.T.);
#10860=ORIENTED_EDGE('',*,*,#8118,.T.);
#10861=ORIENTED_EDGE('',*,*,#8101,.T.);
#10862=ORIENTED_EDGE('',*,*,#8118,.F.);
#10863=ORIENTED_EDGE('',*,*,#8117,.F.);
#10864=ORIENTED_EDGE('',*,*,#8119,.T.);
#10865=ORIENTED_EDGE('',*,*,#8120,.F.);
#10866=ORIENTED_EDGE('',*,*,#8121,.F.);
#10867=ORIENTED_EDGE('',*,*,#8122,.F.);
#10868=ORIENTED_EDGE('',*,*,#8123,.T.);
#10869=ORIENTED_EDGE('',*,*,#8124,.F.);
#10870=ORIENTED_EDGE('',*,*,#8125,.F.);
#10871=ORIENTED_EDGE('',*,*,#8126,.F.);
#10872=ORIENTED_EDGE('',*,*,#8127,.F.);
#10873=ORIENTED_EDGE('',*,*,#8128,.F.);
#10874=ORIENTED_EDGE('',*,*,#8129,.T.);
#10875=ORIENTED_EDGE('',*,*,#8130,.F.);
#10876=ORIENTED_EDGE('',*,*,#8131,.F.);
#10877=ORIENTED_EDGE('',*,*,#8132,.F.);
#10878=ORIENTED_EDGE('',*,*,#8119,.F.);
#10879=ORIENTED_EDGE('',*,*,#8133,.T.);
#10880=ORIENTED_EDGE('',*,*,#8134,.T.);
#10881=ORIENTED_EDGE('',*,*,#8102,.T.);
#10882=ORIENTED_EDGE('',*,*,#8134,.F.);
#10883=ORIENTED_EDGE('',*,*,#8133,.F.);
#10884=ORIENTED_EDGE('',*,*,#8135,.T.);
#10885=ORIENTED_EDGE('',*,*,#8136,.F.);
#10886=ORIENTED_EDGE('',*,*,#8137,.F.);
#10887=ORIENTED_EDGE('',*,*,#8138,.F.);
#10888=ORIENTED_EDGE('',*,*,#8139,.T.);
#10889=ORIENTED_EDGE('',*,*,#8140,.F.);
#10890=ORIENTED_EDGE('',*,*,#8141,.F.);
#10891=ORIENTED_EDGE('',*,*,#8142,.F.);
#10892=ORIENTED_EDGE('',*,*,#8143,.F.);
#10893=ORIENTED_EDGE('',*,*,#8144,.F.);
#10894=ORIENTED_EDGE('',*,*,#8145,.T.);
#10895=ORIENTED_EDGE('',*,*,#8146,.F.);
#10896=ORIENTED_EDGE('',*,*,#8147,.F.);
#10897=ORIENTED_EDGE('',*,*,#8148,.F.);
#10898=ORIENTED_EDGE('',*,*,#8135,.F.);
#10899=ORIENTED_EDGE('',*,*,#8149,.F.);
#10900=ORIENTED_EDGE('',*,*,#8139,.F.);
#10901=ORIENTED_EDGE('',*,*,#8150,.F.);
#10902=ORIENTED_EDGE('',*,*,#8145,.F.);
#10903=ORIENTED_EDGE('',*,*,#8151,.F.);
#10904=ORIENTED_EDGE('',*,*,#8123,.F.);
#10905=ORIENTED_EDGE('',*,*,#8152,.F.);
#10906=ORIENTED_EDGE('',*,*,#8129,.F.);
#10907=ORIENTED_EDGE('',*,*,#8153,.F.);
#10908=ORIENTED_EDGE('',*,*,#8107,.F.);
#10909=ORIENTED_EDGE('',*,*,#8154,.F.);
#10910=ORIENTED_EDGE('',*,*,#8113,.F.);
#10911=ORIENTED_EDGE('',*,*,#8146,.T.);
#10912=ORIENTED_EDGE('',*,*,#8150,.T.);
#10913=ORIENTED_EDGE('',*,*,#8144,.T.);
#10914=ORIENTED_EDGE('',*,*,#8155,.T.);
#10915=ORIENTED_EDGE('',*,*,#8130,.T.);
#10916=ORIENTED_EDGE('',*,*,#8152,.T.);
#10917=ORIENTED_EDGE('',*,*,#8128,.T.);
#10918=ORIENTED_EDGE('',*,*,#8156,.T.);
#10919=ORIENTED_EDGE('',*,*,#8114,.T.);
#10920=ORIENTED_EDGE('',*,*,#8154,.T.);
#10921=ORIENTED_EDGE('',*,*,#8112,.T.);
#10922=ORIENTED_EDGE('',*,*,#8157,.T.);
#10923=ORIENTED_EDGE('',*,*,#8059,.F.);
#10924=ORIENTED_EDGE('',*,*,#8158,.F.);
#10925=ORIENTED_EDGE('',*,*,#8084,.F.);
#10926=ORIENTED_EDGE('',*,*,#8159,.T.);
#10927=ORIENTED_EDGE('',*,*,#8111,.T.);
#10928=ORIENTED_EDGE('',*,*,#8160,.T.);
#10929=ORIENTED_EDGE('',*,*,#8060,.F.);
#10930=ORIENTED_EDGE('',*,*,#8157,.F.);
#10931=ORIENTED_EDGE('',*,*,#8127,.T.);
#10932=ORIENTED_EDGE('',*,*,#8161,.T.);
#10933=ORIENTED_EDGE('',*,*,#8115,.T.);
#10934=ORIENTED_EDGE('',*,*,#8156,.F.);
#10935=ORIENTED_EDGE('',*,*,#8143,.T.);
#10936=ORIENTED_EDGE('',*,*,#8162,.T.);
#10937=ORIENTED_EDGE('',*,*,#8131,.T.);
#10938=ORIENTED_EDGE('',*,*,#8155,.F.);
#10939=ORIENTED_EDGE('',*,*,#8110,.T.);
#10940=ORIENTED_EDGE('',*,*,#8163,.T.);
#10941=ORIENTED_EDGE('',*,*,#8061,.F.);
#10942=ORIENTED_EDGE('',*,*,#8160,.F.);
#10943=ORIENTED_EDGE('',*,*,#8126,.T.);
#10944=ORIENTED_EDGE('',*,*,#8164,.T.);
#10945=ORIENTED_EDGE('',*,*,#8104,.T.);
#10946=ORIENTED_EDGE('',*,*,#8116,.T.);
#10947=ORIENTED_EDGE('',*,*,#8161,.F.);
#10948=ORIENTED_EDGE('',*,*,#8142,.T.);
#10949=ORIENTED_EDGE('',*,*,#8165,.T.);
#10950=ORIENTED_EDGE('',*,*,#8120,.T.);
#10951=ORIENTED_EDGE('',*,*,#8132,.T.);
#10952=ORIENTED_EDGE('',*,*,#8162,.F.);
#10953=ORIENTED_EDGE('',*,*,#8109,.T.);
#10954=ORIENTED_EDGE('',*,*,#8166,.T.);
#10955=ORIENTED_EDGE('',*,*,#8062,.F.);
#10956=ORIENTED_EDGE('',*,*,#8163,.F.);
#10957=ORIENTED_EDGE('',*,*,#8125,.T.);
#10958=ORIENTED_EDGE('',*,*,#8167,.T.);
#10959=ORIENTED_EDGE('',*,*,#8105,.T.);
#10960=ORIENTED_EDGE('',*,*,#8164,.F.);
#10961=ORIENTED_EDGE('',*,*,#8141,.T.);
#10962=ORIENTED_EDGE('',*,*,#8168,.T.);
#10963=ORIENTED_EDGE('',*,*,#8121,.T.);
#10964=ORIENTED_EDGE('',*,*,#8165,.F.);
#10965=ORIENTED_EDGE('',*,*,#8169,.T.);
#10966=ORIENTED_EDGE('',*,*,#8051,.T.);
#10967=ORIENTED_EDGE('',*,*,#8170,.T.);
#10968=ORIENTED_EDGE('',*,*,#8171,.T.);
#10969=ORIENTED_EDGE('',*,*,#8171,.F.);
#10970=ORIENTED_EDGE('',*,*,#8172,.F.);
#10971=ORIENTED_EDGE('',*,*,#8173,.F.);
#10972=ORIENTED_EDGE('',*,*,#8174,.F.);
#10973=ORIENTED_EDGE('',*,*,#8170,.F.);
#10974=ORIENTED_EDGE('',*,*,#8067,.T.);
#10975=ORIENTED_EDGE('',*,*,#8175,.T.);
#10976=ORIENTED_EDGE('',*,*,#8076,.T.);
#10977=ORIENTED_EDGE('',*,*,#8176,.F.);
#10978=ORIENTED_EDGE('',*,*,#8172,.T.);
#10979=ORIENTED_EDGE('',*,*,#8177,.T.);
#10980=ORIENTED_EDGE('',*,*,#8055,.T.);
#10981=ORIENTED_EDGE('',*,*,#8178,.T.);
#10982=ORIENTED_EDGE('',*,*,#8179,.T.);
#10983=ORIENTED_EDGE('',*,*,#8177,.F.);
#10984=ORIENTED_EDGE('',*,*,#8180,.T.);
#10985=ORIENTED_EDGE('',*,*,#8181,.F.);
#10986=ORIENTED_EDGE('',*,*,#8087,.T.);
#10987=ORIENTED_EDGE('',*,*,#8182,.T.);
#10988=ORIENTED_EDGE('',*,*,#8056,.T.);
#10989=ORIENTED_EDGE('',*,*,#8179,.F.);
#10990=ORIENTED_EDGE('',*,*,#8183,.F.);
#10991=ORIENTED_EDGE('',*,*,#8184,.F.);
#10992=ORIENTED_EDGE('',*,*,#8180,.F.);
#10993=ORIENTED_EDGE('',*,*,#8176,.T.);
#10994=ORIENTED_EDGE('',*,*,#8075,.T.);
#10995=ORIENTED_EDGE('',*,*,#8185,.T.);
#10996=ORIENTED_EDGE('',*,*,#8173,.T.);
#10997=ORIENTED_EDGE('',*,*,#8186,.T.);
#10998=ORIENTED_EDGE('',*,*,#8088,.T.);
#10999=ORIENTED_EDGE('',*,*,#8181,.T.);
#11000=ORIENTED_EDGE('',*,*,#8184,.T.);
#11001=ORIENTED_EDGE('',*,*,#8058,.T.);
#11002=ORIENTED_EDGE('',*,*,#8187,.T.);
#11003=ORIENTED_EDGE('',*,*,#8085,.T.);
#11004=ORIENTED_EDGE('',*,*,#8158,.T.);
#11005=ORIENTED_EDGE('',*,*,#8187,.F.);
#11006=ORIENTED_EDGE('',*,*,#8057,.F.);
#11007=ORIENTED_EDGE('',*,*,#8182,.F.);
#11008=ORIENTED_EDGE('',*,*,#8086,.F.);
#11009=ORIENTED_EDGE('',*,*,#8064,.T.);
#11010=ORIENTED_EDGE('',*,*,#8188,.T.);
#11011=ORIENTED_EDGE('',*,*,#8079,.T.);
#11012=ORIENTED_EDGE('',*,*,#8189,.T.);
#11013=ORIENTED_EDGE('',*,*,#8138,.T.);
#11014=ORIENTED_EDGE('',*,*,#8190,.F.);
#11015=ORIENTED_EDGE('',*,*,#8080,.F.);
#11016=ORIENTED_EDGE('',*,*,#8188,.F.);
#11017=ORIENTED_EDGE('',*,*,#8063,.F.);
#11018=ORIENTED_EDGE('',*,*,#8166,.F.);
#11019=ORIENTED_EDGE('',*,*,#8108,.T.);
#11020=ORIENTED_EDGE('',*,*,#8153,.T.);
#11021=ORIENTED_EDGE('',*,*,#8106,.T.);
#11022=ORIENTED_EDGE('',*,*,#8167,.F.);
#11023=ORIENTED_EDGE('',*,*,#8124,.T.);
#11024=ORIENTED_EDGE('',*,*,#8151,.T.);
#11025=ORIENTED_EDGE('',*,*,#8122,.T.);
#11026=ORIENTED_EDGE('',*,*,#8168,.F.);
#11027=ORIENTED_EDGE('',*,*,#8140,.T.);
#11028=ORIENTED_EDGE('',*,*,#8149,.T.);
#11029=ORIENTED_EDGE('',*,*,#8169,.F.);
#11030=ORIENTED_EDGE('',*,*,#8174,.T.);
#11031=ORIENTED_EDGE('',*,*,#8185,.F.);
#11032=ORIENTED_EDGE('',*,*,#8091,.T.);
#11033=ORIENTED_EDGE('',*,*,#8099,.T.);
#11034=ORIENTED_EDGE('',*,*,#8052,.T.);
#11035=ORIENTED_EDGE('',*,*,#8178,.F.);
#11036=ORIENTED_EDGE('',*,*,#8054,.T.);
#11037=ORIENTED_EDGE('',*,*,#8100,.T.);
#11038=ORIENTED_EDGE('',*,*,#8089,.T.);
#11039=ORIENTED_EDGE('',*,*,#8186,.F.);
#11040=ORIENTED_EDGE('',*,*,#8183,.T.);
#11041=ORIENTED_EDGE('',*,*,#8189,.F.);
#11042=ORIENTED_EDGE('',*,*,#8078,.F.);
#11043=ORIENTED_EDGE('',*,*,#8077,.F.);
#11044=ORIENTED_EDGE('',*,*,#8175,.F.);
#11045=ORIENTED_EDGE('',*,*,#8066,.F.);
#11046=ORIENTED_EDGE('',*,*,#8065,.F.);
#11047=ORIENTED_EDGE('',*,*,#8137,.T.);
#11048=ORIENTED_EDGE('',*,*,#8191,.F.);
#11049=ORIENTED_EDGE('',*,*,#8081,.F.);
#11050=ORIENTED_EDGE('',*,*,#8190,.T.);
#11051=ORIENTED_EDGE('',*,*,#8136,.T.);
#11052=ORIENTED_EDGE('',*,*,#8148,.T.);
#11053=ORIENTED_EDGE('',*,*,#8192,.F.);
#11054=ORIENTED_EDGE('',*,*,#8082,.F.);
#11055=ORIENTED_EDGE('',*,*,#8191,.T.);
#11056=ORIENTED_EDGE('',*,*,#8147,.T.);
#11057=ORIENTED_EDGE('',*,*,#8159,.F.);
#11058=ORIENTED_EDGE('',*,*,#8083,.F.);
#11059=ORIENTED_EDGE('',*,*,#8192,.T.);
#14310=CONICAL_SURFACE('',#15615,1.65,0.785398163397459);
#14311=CONICAL_SURFACE('',#15622,0.775000000000001,1.02974425867665);
#14312=CONICAL_SURFACE('',#15623,1.65,0.785398163397448);
#14313=CONICAL_SURFACE('',#15630,1.55,1.02974425867665);
#14314=CONICAL_SURFACE('',#15631,2.7,0.785398163397441);
#14315=CONICAL_SURFACE('',#15647,2.7,0.785398163397441);
#14316=CONICAL_SURFACE('',#15659,2.7,0.785398163397456);
#14549=ADVANCED_FACE('',(#1814),#14310,.F.);
#14550=ADVANCED_FACE('',(#1815),#1283,.T.);
#14551=ADVANCED_FACE('',(#1816),#915,.F.);
#14552=ADVANCED_FACE('',(#1817),#14311,.F.);
#14553=ADVANCED_FACE('',(#1818),#14312,.F.);
#14554=ADVANCED_FACE('',(#1819),#1284,.F.);
#14555=ADVANCED_FACE('',(#1820),#916,.F.);
#14556=ADVANCED_FACE('',(#1821),#14313,.F.);
#14557=ADVANCED_FACE('',(#1822),#14314,.F.);
#14558=ADVANCED_FACE('',(#1823,#1169,#1170,#1171),#1285,.T.);
#14559=ADVANCED_FACE('',(#1824),#917,.F.);
#14560=ADVANCED_FACE('',(#1825),#14315,.F.);
#14561=ADVANCED_FACE('',(#1826),#918,.F.);
#14562=ADVANCED_FACE('',(#1827),#14316,.F.);
#14563=ADVANCED_FACE('',(#1828),#919,.F.);
#14564=ADVANCED_FACE('',(#1829),#1286,.F.);
#14565=ADVANCED_FACE('',(#1830),#1287,.F.);
#14566=ADVANCED_FACE('',(#1831),#1288,.F.);
#14567=ADVANCED_FACE('',(#1832),#1289,.F.);
#14568=ADVANCED_FACE('',(#1833),#1290,.F.);
#14569=ADVANCED_FACE('',(#1834),#1291,.F.);
#14570=ADVANCED_FACE('',(#1835),#1292,.T.);
#14571=ADVANCED_FACE('',(#1836),#1293,.T.);
#14572=ADVANCED_FACE('',(#1837),#1294,.T.);
#14573=ADVANCED_FACE('',(#1838),#1295,.T.);
#14574=ADVANCED_FACE('',(#1839),#1296,.T.);
#14575=ADVANCED_FACE('',(#1840),#1297,.T.);
#14576=ADVANCED_FACE('',(#1841),#1298,.T.);
#14577=ADVANCED_FACE('',(#1842),#1299,.T.);
#14578=ADVANCED_FACE('',(#1843),#1300,.T.);
#14579=ADVANCED_FACE('',(#1844),#1301,.T.);
#14580=ADVANCED_FACE('',(#1845),#1302,.T.);
#14581=ADVANCED_FACE('',(#1846),#1303,.T.);
#14582=ADVANCED_FACE('',(#1847),#1304,.T.);
#14583=ADVANCED_FACE('',(#1848),#1305,.T.);
#14584=ADVANCED_FACE('',(#1849),#1306,.T.);
#14585=ADVANCED_FACE('',(#1850),#1307,.T.);
#14586=ADVANCED_FACE('',(#1851),#1308,.T.);
#14587=ADVANCED_FACE('',(#1852),#1309,.T.);
#14588=ADVANCED_FACE('',(#1853),#1310,.T.);
#14589=ADVANCED_FACE('',(#1854),#1311,.T.);
#14590=ADVANCED_FACE('',(#1855),#1312,.T.);
#14591=ADVANCED_FACE('',(#1856),#1313,.T.);
#14592=ADVANCED_FACE('',(#1857),#1314,.T.);
#14593=ADVANCED_FACE('',(#1858),#1315,.T.);
#14594=ADVANCED_FACE('',(#1859),#1316,.T.);
#14595=ADVANCED_FACE('',(#1860),#1317,.T.);
#14596=ADVANCED_FACE('',(#1861),#1318,.T.);
#14597=ADVANCED_FACE('',(#1862),#1319,.T.);
#15086=CLOSED_SHELL('',(#14549,#14550,#14551,#14552,#14553,#14554,#14555,
#14556,#14557,#14558,#14559,#14560,#14561,#14562,#14563,#14564,#14565,#14566,
#14567,#14568,#14569,#14570,#14571,#14572,#14573,#14574,#14575,#14576,#14577,
#14578,#14579,#14580,#14581,#14582,#14583,#14584,#14585,#14586,#14587,#14588,
#14589,#14590,#14591,#14592,#14593,#14594,#14595,#14596,#14597));
#15614=AXIS2_PLACEMENT_3D('',#21617,#17728,#17729);
#15615=AXIS2_PLACEMENT_3D('',#21618,#17730,#17731);
#15616=AXIS2_PLACEMENT_3D('',#21620,#17732,#17733);
#15617=AXIS2_PLACEMENT_3D('',#21623,#17735,#17736);
#15618=AXIS2_PLACEMENT_3D('',#21624,#17737,#17738);
#15619=AXIS2_PLACEMENT_3D('',#21658,#17756,#17757);
#15620=AXIS2_PLACEMENT_3D('',#21662,#17759,#17760);
#15621=AXIS2_PLACEMENT_3D('',#21663,#17761,#17762);
#15622=AXIS2_PLACEMENT_3D('',#21664,#17763,#17764);
#15623=AXIS2_PLACEMENT_3D('',#21667,#17766,#17767);
#15624=AXIS2_PLACEMENT_3D('',#21669,#17768,#17769);
#15625=AXIS2_PLACEMENT_3D('',#21672,#17771,#17772);
#15626=AXIS2_PLACEMENT_3D('',#21673,#17773,#17774);
#15627=AXIS2_PLACEMENT_3D('',#21707,#17792,#17793);
#15628=AXIS2_PLACEMENT_3D('',#21711,#17795,#17796);
#15629=AXIS2_PLACEMENT_3D('',#21712,#17797,#17798);
#15630=AXIS2_PLACEMENT_3D('',#21713,#17799,#17800);
#15631=AXIS2_PLACEMENT_3D('',#21716,#17802,#17803);
#15632=AXIS2_PLACEMENT_3D('',#21718,#17804,#17805);
#15633=AXIS2_PLACEMENT_3D('',#21721,#17807,#17808);
#15634=AXIS2_PLACEMENT_3D('',#21722,#17809,#17810);
#15635=AXIS2_PLACEMENT_3D('',#21726,#17813,#17814);
#15636=AXIS2_PLACEMENT_3D('',#21728,#17815,#17816);
#15637=AXIS2_PLACEMENT_3D('',#21729,#17817,#17818);
#15638=AXIS2_PLACEMENT_3D('',#21733,#17820,#17821);
#15639=AXIS2_PLACEMENT_3D('',#21737,#17823,#17824);
#15640=AXIS2_PLACEMENT_3D('',#21739,#17825,#17826);
#15641=AXIS2_PLACEMENT_3D('',#21741,#17827,#17828);
#15642=AXIS2_PLACEMENT_3D('',#21745,#17830,#17831);
#15643=AXIS2_PLACEMENT_3D('',#21749,#17833,#17834);
#15644=AXIS2_PLACEMENT_3D('',#21751,#17835,#17836);
#15645=AXIS2_PLACEMENT_3D('',#21753,#17837,#17838);
#15646=AXIS2_PLACEMENT_3D('',#21756,#17840,#17841);
#15647=AXIS2_PLACEMENT_3D('',#21757,#17842,#17843);
#15648=AXIS2_PLACEMENT_3D('',#21759,#17844,#17845);
#15649=AXIS2_PLACEMENT_3D('',#21761,#17847,#17848);
#15650=AXIS2_PLACEMENT_3D('',#21765,#17850,#17851);
#15651=AXIS2_PLACEMENT_3D('',#21769,#17853,#17854);
#15652=AXIS2_PLACEMENT_3D('',#21771,#17855,#17856);
#15653=AXIS2_PLACEMENT_3D('',#21773,#17857,#17858);
#15654=AXIS2_PLACEMENT_3D('',#21777,#17860,#17861);
#15655=AXIS2_PLACEMENT_3D('',#21781,#17863,#17864);
#15656=AXIS2_PLACEMENT_3D('',#21783,#17865,#17866);
#15657=AXIS2_PLACEMENT_3D('',#21785,#17867,#17868);
#15658=AXIS2_PLACEMENT_3D('',#21788,#17870,#17871);
#15659=AXIS2_PLACEMENT_3D('',#21789,#17872,#17873);
#15660=AXIS2_PLACEMENT_3D('',#21791,#17874,#17875);
#15661=AXIS2_PLACEMENT_3D('',#21793,#17877,#17878);
#15662=AXIS2_PLACEMENT_3D('',#21797,#17880,#17881);
#15663=AXIS2_PLACEMENT_3D('',#21801,#17883,#17884);
#15664=AXIS2_PLACEMENT_3D('',#21803,#17885,#17886);
#15665=AXIS2_PLACEMENT_3D('',#21805,#17887,#17888);
#15666=AXIS2_PLACEMENT_3D('',#21809,#17890,#17891);
#15667=AXIS2_PLACEMENT_3D('',#21813,#17893,#17894);
#15668=AXIS2_PLACEMENT_3D('',#21815,#17895,#17896);
#15669=AXIS2_PLACEMENT_3D('',#21817,#17897,#17898);
#15670=AXIS2_PLACEMENT_3D('',#21820,#17900,#17901);
#15671=AXIS2_PLACEMENT_3D('',#21821,#17902,#17903);
#15672=AXIS2_PLACEMENT_3D('',#21823,#17905,#17906);
#15673=AXIS2_PLACEMENT_3D('',#21825,#17908,#17909);
#15674=AXIS2_PLACEMENT_3D('',#21827,#17911,#17912);
#15675=AXIS2_PLACEMENT_3D('',#21829,#17914,#17915);
#15676=AXIS2_PLACEMENT_3D('',#21831,#17917,#17918);
#15677=AXIS2_PLACEMENT_3D('',#21833,#17920,#17921);
#15678=AXIS2_PLACEMENT_3D('',#21839,#17927,#17928);
#15679=AXIS2_PLACEMENT_3D('',#21841,#17930,#17931);
#15680=AXIS2_PLACEMENT_3D('',#21843,#17933,#17934);
#15681=AXIS2_PLACEMENT_3D('',#21845,#17936,#17937);
#15682=AXIS2_PLACEMENT_3D('',#21847,#17939,#17940);
#15683=AXIS2_PLACEMENT_3D('',#21849,#17942,#17943);
#15684=AXIS2_PLACEMENT_3D('',#21851,#17945,#17946);
#15685=AXIS2_PLACEMENT_3D('',#21853,#17948,#17949);
#15686=AXIS2_PLACEMENT_3D('',#21855,#17951,#17952);
#15687=AXIS2_PLACEMENT_3D('',#21857,#17954,#17955);
#15688=AXIS2_PLACEMENT_3D('',#21863,#17959,#17960);
#15689=AXIS2_PLACEMENT_3D('',#21869,#17964,#17965);
#15690=AXIS2_PLACEMENT_3D('',#21872,#17968,#17969);
#15691=AXIS2_PLACEMENT_3D('',#21878,#17973,#17974);
#15692=AXIS2_PLACEMENT_3D('',#21883,#17978,#17979);
#15693=AXIS2_PLACEMENT_3D('',#21887,#17982,#17983);
#15694=AXIS2_PLACEMENT_3D('',#21889,#17985,#17986);
#15695=AXIS2_PLACEMENT_3D('',#21891,#17988,#17989);
#15696=AXIS2_PLACEMENT_3D('',#21893,#17991,#17992);
#15697=AXIS2_PLACEMENT_3D('',#21894,#17993,#17994);
#15698=AXIS2_PLACEMENT_3D('',#21897,#17997,#17998);
#15699=AXIS2_PLACEMENT_3D('',#21899,#18000,#18001);
#15700=AXIS2_PLACEMENT_3D('',#21900,#18002,#18003);
#15701=AXIS2_PLACEMENT_3D('',#21901,#18004,#18005);
#15702=AXIS2_PLACEMENT_3D('',#21902,#18006,#18007);
#15703=AXIS2_PLACEMENT_3D('',#21904,#18009,#18010);
#15704=AXIS2_PLACEMENT_3D('',#21906,#18012,#18013);
#17728=DIRECTION('axis',(0.,0.,1.));
#17729=DIRECTION('refdir',(1.,0.,0.));
#17730=DIRECTION('center_axis',(1.,0.,0.));
#17731=DIRECTION('ref_axis',(0.,0.,-1.));
#17732=DIRECTION('center_axis',(-1.,0.,0.));
#17733=DIRECTION('ref_axis',(0.,0.,-1.));
#17734=DIRECTION('',(0.70710678118654,-8.65956056235502E-17,0.707106781186555));
#17735=DIRECTION('center_axis',(1.,0.,0.));
#17736=DIRECTION('ref_axis',(0.,0.,-1.));
#17737=DIRECTION('center_axis',(1.,0.,0.));
#17738=DIRECTION('ref_axis',(0.,0.,-1.));
#17739=DIRECTION('',(0.,0.,1.));
#17740=DIRECTION('',(0.,-0.70710678118655,0.707106781186545));
#17741=DIRECTION('',(0.,1.,0.));
#17742=DIRECTION('',(0.,-0.707106781186547,-0.707106781186547));
#17743=DIRECTION('',(0.,0.,-1.));
#17744=DIRECTION('',(0.,0.707106781186547,-0.707106781186547));
#17745=DIRECTION('',(0.,-1.,0.));
#17746=DIRECTION('',(0.,0.923879532511291,0.38268343236508));
#17747=DIRECTION('',(0.,-0.707106781186547,-0.707106781186547));
#17748=DIRECTION('',(0.,0.,-1.));
#17749=DIRECTION('',(0.,-1.,0.));
#17750=DIRECTION('',(0.,0.,1.));
#17751=DIRECTION('',(0.,-0.707106781186548,0.707106781186547));
#17752=DIRECTION('',(0.,0.923879532511287,-0.38268343236509));
#17753=DIRECTION('',(0.,-1.,0.));
#17754=DIRECTION('',(0.,-1.,0.));
#17755=DIRECTION('',(0.,0.707106781186549,0.707106781186546));
#17756=DIRECTION('center_axis',(-1.,0.,0.));
#17757=DIRECTION('ref_axis',(0.,0.,-1.));
#17758=DIRECTION('',(-1.,0.,0.));
#17759=DIRECTION('center_axis',(-1.,0.,0.));
#17760=DIRECTION('ref_axis',(0.,0.,-1.));
#17761=DIRECTION('center_axis',(-1.,0.,0.));
#17762=DIRECTION('ref_axis',(0.,0.,-1.));
#17763=DIRECTION('center_axis',(1.,0.,0.));
#17764=DIRECTION('ref_axis',(0.,1.,0.));
#17765=DIRECTION('',(0.515038074910058,-0.85716730070211,-1.04972719113862E-16));
#17766=DIRECTION('center_axis',(-1.,0.,0.));
#17767=DIRECTION('ref_axis',(0.,0.,-1.));
#17768=DIRECTION('center_axis',(1.,0.,0.));
#17769=DIRECTION('ref_axis',(0.,0.,-1.));
#17770=DIRECTION('',(-0.707106781186548,8.65956056235493E-17,0.707106781186547));
#17771=DIRECTION('center_axis',(-1.,0.,0.));
#17772=DIRECTION('ref_axis',(0.,0.,-1.));
#17773=DIRECTION('center_axis',(1.,0.,0.));
#17774=DIRECTION('ref_axis',(0.,0.,-1.));
#17775=DIRECTION('',(0.,0.,-1.));
#17776=DIRECTION('',(0.,-0.707106781186549,-0.707106781186546));
#17777=DIRECTION('',(0.,1.,0.));
#17778=DIRECTION('',(0.,1.,0.));
#17779=DIRECTION('',(0.,-0.923879532511287,0.38268343236509));
#17780=DIRECTION('',(0.,0.707106781186548,-0.707106781186547));
#17781=DIRECTION('',(0.,0.,-1.));
#17782=DIRECTION('',(0.,1.,0.));
#17783=DIRECTION('',(0.,0.,1.));
#17784=DIRECTION('',(0.,0.707106781186547,0.707106781186547));
#17785=DIRECTION('',(0.,-0.923879532511291,-0.38268343236508));
#17786=DIRECTION('',(0.,1.,0.));
#17787=DIRECTION('',(0.,-0.707106781186547,0.707106781186547));
#17788=DIRECTION('',(0.,0.,1.));
#17789=DIRECTION('',(0.,0.707106781186547,0.707106781186547));
#17790=DIRECTION('',(0.,-1.,0.));
#17791=DIRECTION('',(0.,0.70710678118655,-0.707106781186545));
#17792=DIRECTION('center_axis',(1.,0.,0.));
#17793=DIRECTION('ref_axis',(0.,0.,-1.));
#17794=DIRECTION('',(1.,0.,0.));
#17795=DIRECTION('center_axis',(1.,0.,0.));
#17796=DIRECTION('ref_axis',(0.,0.,-1.));
#17797=DIRECTION('center_axis',(1.,0.,0.));
#17798=DIRECTION('ref_axis',(0.,0.,-1.));
#17799=DIRECTION('center_axis',(-1.,0.,0.));
#17800=DIRECTION('ref_axis',(0.,1.,0.));
#17801=DIRECTION('',(-0.515038074910058,-0.85716730070211,1.04972719113862E-16));
#17802=DIRECTION('center_axis',(0.,0.,-1.));
#17803=DIRECTION('ref_axis',(1.,0.,0.));
#17804=DIRECTION('center_axis',(0.,0.,1.));
#17805=DIRECTION('ref_axis',(1.,0.,0.));
#17806=DIRECTION('',(-0.707106781186542,8.65956056235487E-17,-0.707106781186553));
#17807=DIRECTION('center_axis',(0.,0.,-1.));
#17808=DIRECTION('ref_axis',(1.,0.,0.));
#17809=DIRECTION('center_axis',(0.,0.,-1.));
#17810=DIRECTION('ref_axis',(0.,1.,0.));
#17811=DIRECTION('',(1.,0.,0.));
#17812=DIRECTION('',(-1.,0.,0.));
#17813=DIRECTION('center_axis',(0.,0.,-1.));
#17814=DIRECTION('ref_axis',(1.,0.,0.));
#17815=DIRECTION('center_axis',(0.,0.,-1.));
#17816=DIRECTION('ref_axis',(1.,0.,0.));
#17817=DIRECTION('center_axis',(0.,0.,1.));
#17818=DIRECTION('ref_axis',(1.,0.,0.));
#17819=DIRECTION('',(0.,0.,1.));
#17820=DIRECTION('center_axis',(0.,0.,-1.));
#17821=DIRECTION('ref_axis',(1.,0.,0.));
#17822=DIRECTION('',(0.,0.,-1.));
#17823=DIRECTION('center_axis',(0.,-0.707106781186547,-0.707106781186548));
#17824=DIRECTION('ref_axis',(0.,0.707106781186548,-0.707106781186547));
#17825=DIRECTION('center_axis',(0.,0.,1.));
#17826=DIRECTION('ref_axis',(1.,0.,0.));
#17827=DIRECTION('center_axis',(0.,-0.707106781186547,-0.707106781186548));
#17828=DIRECTION('ref_axis',(0.,0.707106781186548,-0.707106781186547));
#17829=DIRECTION('',(0.,0.,1.));
#17830=DIRECTION('center_axis',(0.,0.,-1.));
#17831=DIRECTION('ref_axis',(1.,0.,0.));
#17832=DIRECTION('',(0.,0.,-1.));
#17833=DIRECTION('center_axis',(0.,0.707106781186548,-0.707106781186548));
#17834=DIRECTION('ref_axis',(0.,0.707106781186547,0.707106781186547));
#17835=DIRECTION('center_axis',(0.,0.,1.));
#17836=DIRECTION('ref_axis',(1.,0.,0.));
#17837=DIRECTION('center_axis',(0.,0.707106781186548,-0.707106781186548));
#17838=DIRECTION('ref_axis',(0.,0.707106781186547,0.707106781186547));
#17839=DIRECTION('',(0.,0.,1.));
#17840=DIRECTION('center_axis',(0.,0.,-1.));
#17841=DIRECTION('ref_axis',(1.,0.,0.));
#17842=DIRECTION('center_axis',(0.,0.,-1.));
#17843=DIRECTION('ref_axis',(1.,0.,0.));
#17844=DIRECTION('center_axis',(0.,0.,1.));
#17845=DIRECTION('ref_axis',(1.,0.,0.));
#17846=DIRECTION('',(-0.707106781186542,8.65956056235487E-17,-0.707106781186553));
#17847=DIRECTION('center_axis',(0.,0.,1.));
#17848=DIRECTION('ref_axis',(1.,0.,0.));
#17849=DIRECTION('',(0.,0.,1.));
#17850=DIRECTION('center_axis',(0.,0.,-1.));
#17851=DIRECTION('ref_axis',(1.,0.,0.));
#17852=DIRECTION('',(0.,0.,-1.));
#17853=DIRECTION('center_axis',(0.,-0.707106781186547,-0.707106781186548));
#17854=DIRECTION('ref_axis',(0.,0.707106781186548,-0.707106781186547));
#17855=DIRECTION('center_axis',(0.,0.,1.));
#17856=DIRECTION('ref_axis',(1.,0.,0.));
#17857=DIRECTION('center_axis',(0.,-0.707106781186547,-0.707106781186548));
#17858=DIRECTION('ref_axis',(0.,0.707106781186548,-0.707106781186547));
#17859=DIRECTION('',(0.,0.,1.));
#17860=DIRECTION('center_axis',(0.,0.,-1.));
#17861=DIRECTION('ref_axis',(1.,0.,0.));
#17862=DIRECTION('',(0.,0.,-1.));
#17863=DIRECTION('center_axis',(0.,0.707106781186548,-0.707106781186548));
#17864=DIRECTION('ref_axis',(0.,0.707106781186547,0.707106781186547));
#17865=DIRECTION('center_axis',(0.,0.,1.));
#17866=DIRECTION('ref_axis',(1.,0.,0.));
#17867=DIRECTION('center_axis',(0.,0.707106781186548,-0.707106781186548));
#17868=DIRECTION('ref_axis',(0.,0.707106781186547,0.707106781186547));
#17869=DIRECTION('',(0.,0.,1.));
#17870=DIRECTION('center_axis',(0.,0.,-1.));
#17871=DIRECTION('ref_axis',(1.,0.,0.));
#17872=DIRECTION('center_axis',(0.,0.,-1.));
#17873=DIRECTION('ref_axis',(1.,0.,0.));
#17874=DIRECTION('center_axis',(0.,0.,1.));
#17875=DIRECTION('ref_axis',(1.,0.,0.));
#17876=DIRECTION('',(-0.707106781186553,8.659560562355E-17,-0.707106781186542));
#17877=DIRECTION('center_axis',(0.,0.,1.));
#17878=DIRECTION('ref_axis',(1.,0.,0.));
#17879=DIRECTION('',(0.,0.,1.));
#17880=DIRECTION('center_axis',(0.,0.,-1.));
#17881=DIRECTION('ref_axis',(1.,0.,0.));
#17882=DIRECTION('',(0.,0.,-1.));
#17883=DIRECTION('center_axis',(0.,-0.707106781186547,-0.707106781186548));
#17884=DIRECTION('ref_axis',(0.,0.707106781186548,-0.707106781186547));
#17885=DIRECTION('center_axis',(0.,0.,1.));
#17886=DIRECTION('ref_axis',(1.,0.,0.));
#17887=DIRECTION('center_axis',(0.,-0.707106781186547,-0.707106781186548));
#17888=DIRECTION('ref_axis',(0.,0.707106781186548,-0.707106781186547));
#17889=DIRECTION('',(0.,0.,1.));
#17890=DIRECTION('center_axis',(0.,0.,-1.));
#17891=DIRECTION('ref_axis',(1.,0.,0.));
#17892=DIRECTION('',(0.,0.,-1.));
#17893=DIRECTION('center_axis',(0.,0.707106781186548,-0.707106781186548));
#17894=DIRECTION('ref_axis',(0.,0.707106781186548,0.707106781186548));
#17895=DIRECTION('center_axis',(0.,0.,1.));
#17896=DIRECTION('ref_axis',(1.,0.,0.));
#17897=DIRECTION('center_axis',(0.,0.707106781186548,-0.707106781186548));
#17898=DIRECTION('ref_axis',(0.,0.707106781186548,0.707106781186548));
#17899=DIRECTION('',(0.,0.,1.));
#17900=DIRECTION('center_axis',(0.,0.,-1.));
#17901=DIRECTION('ref_axis',(1.,0.,0.));
#17902=DIRECTION('center_axis',(0.,0.,1.));
#17903=DIRECTION('ref_axis',(1.,0.,0.));
#17904=DIRECTION('',(-1.,0.,0.));
#17905=DIRECTION('center_axis',(0.,0.,1.));
#17906=DIRECTION('ref_axis',(1.,0.,0.));
#17907=DIRECTION('',(1.,0.,0.));
#17908=DIRECTION('center_axis',(0.,0.,1.));
#17909=DIRECTION('ref_axis',(1.,0.,0.));
#17910=DIRECTION('',(-1.,0.,0.));
#17911=DIRECTION('center_axis',(0.,0.,1.));
#17912=DIRECTION('ref_axis',(1.,0.,0.));
#17913=DIRECTION('',(1.,0.,0.));
#17914=DIRECTION('center_axis',(0.,0.,1.));
#17915=DIRECTION('ref_axis',(1.,0.,0.));
#17916=DIRECTION('',(-1.,0.,0.));
#17917=DIRECTION('center_axis',(0.,0.,1.));
#17918=DIRECTION('ref_axis',(1.,0.,0.));
#17919=DIRECTION('',(1.,0.,0.));
#17920=DIRECTION('center_axis',(0.,-0.707106781186548,0.707106781186548));
#17921=DIRECTION('ref_axis',(0.,-0.707106781186548,-0.707106781186548));
#17922=DIRECTION('',(1.,0.,0.));
#17923=DIRECTION('',(1.,0.,0.));
#17924=DIRECTION('',(1.,0.,0.));
#17925=DIRECTION('',(1.,0.,0.));
#17926=DIRECTION('',(1.,0.,0.));
#17927=DIRECTION('center_axis',(0.,-1.,0.));
#17928=DIRECTION('ref_axis',(0.,0.,-1.));
#17929=DIRECTION('',(1.,0.,0.));
#17930=DIRECTION('center_axis',(0.,-1.,0.));
#17931=DIRECTION('ref_axis',(0.,0.,-1.));
#17932=DIRECTION('',(1.,0.,0.));
#17933=DIRECTION('center_axis',(0.,-1.,0.));
#17934=DIRECTION('ref_axis',(0.,0.,-1.));
#17935=DIRECTION('',(1.,0.,0.));
#17936=DIRECTION('center_axis',(0.,0.,1.));
#17937=DIRECTION('ref_axis',(0.,-1.,0.));
#17938=DIRECTION('',(1.,0.,0.));
#17939=DIRECTION('center_axis',(0.,0.,1.));
#17940=DIRECTION('ref_axis',(0.,-1.,0.));
#17941=DIRECTION('',(1.,0.,0.));
#17942=DIRECTION('center_axis',(0.,0.,1.));
#17943=DIRECTION('ref_axis',(0.,-1.,0.));
#17944=DIRECTION('',(1.,0.,0.));
#17945=DIRECTION('center_axis',(0.,1.,0.));
#17946=DIRECTION('ref_axis',(0.,0.,1.));
#17947=DIRECTION('',(1.,0.,0.));
#17948=DIRECTION('center_axis',(0.,1.,0.));
#17949=DIRECTION('ref_axis',(0.,0.,1.));
#17950=DIRECTION('',(1.,0.,0.));
#17951=DIRECTION('center_axis',(0.,1.,0.));
#17952=DIRECTION('ref_axis',(0.,0.,1.));
#17953=DIRECTION('',(1.,0.,0.));
#17954=DIRECTION('center_axis',(0.707106781186534,-0.707106781186561,0.));
#17955=DIRECTION('ref_axis',(0.,0.,-1.));
#17956=DIRECTION('',(0.577350269189641,0.57735026918962,-0.577350269189616));
#17957=DIRECTION('',(-0.577350269189641,-0.57735026918962,-0.577350269189617));
#17958=DIRECTION('',(0.,0.,-1.));
#17959=DIRECTION('center_axis',(0.,-1.,0.));
#17960=DIRECTION('ref_axis',(0.,0.,-1.));
#17961=DIRECTION('',(1.,0.,0.));
#17962=DIRECTION('',(0.,0.,1.));
#17963=DIRECTION('',(-1.,0.,0.));
#17964=DIRECTION('center_axis',(0.,-0.707106781186546,0.707106781186549));
#17965=DIRECTION('ref_axis',(1.,0.,0.));
#17966=DIRECTION('',(-1.,0.,0.));
#17967=DIRECTION('',(-0.577350269189627,0.577350269189627,0.577350269189624));
#17968=DIRECTION('center_axis',(0.707106781186532,0.707106781186563,0.));
#17969=DIRECTION('ref_axis',(0.,0.,-1.));
#17970=DIRECTION('',(0.577350269189643,-0.577350269189617,0.577350269189617));
#17971=DIRECTION('',(-0.577350269189643,0.577350269189617,0.577350269189617));
#17972=DIRECTION('',(0.,0.,1.));
#17973=DIRECTION('center_axis',(0.,0.707106781186548,0.707106781186548));
#17974=DIRECTION('ref_axis',(1.,0.,0.));
#17975=DIRECTION('',(-1.,0.,0.));
#17976=DIRECTION('',(0.577350269189629,0.577350269189624,-0.577350269189624));
#17977=DIRECTION('',(1.,0.,0.));
#17978=DIRECTION('center_axis',(0.,1.,0.));
#17979=DIRECTION('ref_axis',(0.,0.,1.));
#17980=DIRECTION('',(1.,0.,0.));
#17981=DIRECTION('',(0.,0.,-1.));
#17982=DIRECTION('center_axis',(-0.707106781186548,-0.707106781186548,0.));
#17983=DIRECTION('ref_axis',(0.,0.,1.));
#17984=DIRECTION('',(0.577350269189627,-0.577350269189627,0.577350269189623));
#17985=DIRECTION('center_axis',(-0.707106781186545,0.70710678118655,0.));
#17986=DIRECTION('ref_axis',(0.,0.,1.));
#17987=DIRECTION('',(-0.577350269189629,-0.577350269189624,-0.577350269189624));
#17988=DIRECTION('center_axis',(0.,-0.38268343236508,0.923879532511291));
#17989=DIRECTION('ref_axis',(1.,0.,0.));
#17990=DIRECTION('',(-1.,0.,0.));
#17991=DIRECTION('center_axis',(0.,0.,1.));
#17992=DIRECTION('ref_axis',(0.,-1.,0.));
#17993=DIRECTION('center_axis',(0.,0.38268343236509,0.923879532511287));
#17994=DIRECTION('ref_axis',(1.,0.,0.));
#17995=DIRECTION('',(-1.,0.,0.));
#17996=DIRECTION('',(1.,0.,0.));
#17997=DIRECTION('center_axis',(0.,0.707106781186547,0.707106781186548));
#17998=DIRECTION('ref_axis',(0.,-0.707106781186548,0.707106781186547));
#17999=DIRECTION('',(1.,0.,0.));
#18000=DIRECTION('center_axis',(0.,-0.707106781186545,-0.70710678118655));
#18001=DIRECTION('ref_axis',(-1.,0.,0.));
#18002=DIRECTION('center_axis',(0.,0.707106781186548,-0.707106781186548));
#18003=DIRECTION('ref_axis',(-1.,0.,0.));
#18004=DIRECTION('center_axis',(0.,0.,1.));
#18005=DIRECTION('ref_axis',(0.,-1.,0.));
#18006=DIRECTION('center_axis',(0.,1.,0.));
#18007=DIRECTION('ref_axis',(0.,0.,1.));
#18008=DIRECTION('',(1.,0.,0.));
#18009=DIRECTION('center_axis',(0.,0.,1.));
#18010=DIRECTION('ref_axis',(0.,-1.,0.));
#18011=DIRECTION('',(1.,0.,0.));
#18012=DIRECTION('center_axis',(0.,-1.,0.));
#18013=DIRECTION('ref_axis',(0.,0.,-1.));
#21617=CARTESIAN_POINT('',(0.,0.,0.));
#21618=CARTESIAN_POINT('Origin',(204.9,11.,29.5));
#21619=CARTESIAN_POINT('',(204.8,11.,31.05));
#21620=CARTESIAN_POINT('Origin',(204.8,11.,29.5));
#21621=CARTESIAN_POINT('',(205.,11.,31.25));
#21622=CARTESIAN_POINT('',(204.9,11.,31.15));
#21623=CARTESIAN_POINT('Origin',(205.,11.,29.5));
#21624=CARTESIAN_POINT('Origin',(205.,21.,27.875));
#21625=CARTESIAN_POINT('',(205.,6.3,24.7));
#21626=CARTESIAN_POINT('',(205.,6.3,31.05));
#21627=CARTESIAN_POINT('',(205.,6.3,29.5625));
#21628=CARTESIAN_POINT('',(205.,6.5,24.5));
#21629=CARTESIAN_POINT('',(205.,9.15625000000002,21.84375));
#21630=CARTESIAN_POINT('',(205.,35.5,24.5));
#21631=CARTESIAN_POINT('',(205.,36.,24.5));
#21632=CARTESIAN_POINT('',(205.,35.7,24.7));
#21633=CARTESIAN_POINT('',(205.,32.84375,21.84375));
#21634=CARTESIAN_POINT('',(205.,35.7,31.05));
#21635=CARTESIAN_POINT('',(205.,35.7,26.1875));
#21636=CARTESIAN_POINT('',(205.,35.5,31.25));
#21637=CARTESIAN_POINT('',(205.,32.84375,33.90625));
#21638=CARTESIAN_POINT('',(205.,24.696,31.25));
#21639=CARTESIAN_POINT('',(205.,24.496,31.25));
#21640=CARTESIAN_POINT('',(205.,24.3545786437627,31.1085786437627));
#21641=CARTESIAN_POINT('',(205.,22.4366566484982,30.3141493417505));
#21642=CARTESIAN_POINT('',(205.,21.6,28.354));
#21643=CARTESIAN_POINT('',(205.,21.6,28.354));
#21644=CARTESIAN_POINT('',(205.,21.6,27.154));
#21645=CARTESIAN_POINT('',(205.,21.6,27.154));
#21646=CARTESIAN_POINT('',(205.,20.4,27.154));
#21647=CARTESIAN_POINT('',(205.,20.4,27.154));
#21648=CARTESIAN_POINT('',(205.,20.4,28.354));
#21649=CARTESIAN_POINT('',(205.,20.4,28.354));
#21650=CARTESIAN_POINT('',(205.,17.6454213562373,31.1085786437627));
#21651=CARTESIAN_POINT('',(205.,17.504,31.25));
#21652=CARTESIAN_POINT('',(205.,17.304,31.25));
#21653=CARTESIAN_POINT('',(205.,19.5633433515018,30.3141493417505));
#21654=CARTESIAN_POINT('',(205.,6.,31.25));
#21655=CARTESIAN_POINT('',(205.,6.5,31.25));
#21656=CARTESIAN_POINT('',(205.,6.,31.25));
#21657=CARTESIAN_POINT('',(205.,9.15625000000002,33.90625));
#21658=CARTESIAN_POINT('Origin',(205.,11.,29.5));
#21659=CARTESIAN_POINT('',(198.,11.,31.05));
#21660=CARTESIAN_POINT('',(205.,11.,31.05));
#21661=CARTESIAN_POINT('',(198.,9.45,29.5));
#21662=CARTESIAN_POINT('Origin',(198.,11.,29.5));
#21663=CARTESIAN_POINT('Origin',(198.,11.,29.5));
#21664=CARTESIAN_POINT('Origin',(197.534333020254,11.,29.5));
#21665=CARTESIAN_POINT('',(197.068666040507,11.,29.5));
#21666=CARTESIAN_POINT('',(197.534333020254,10.225,29.5));
#21667=CARTESIAN_POINT('Origin',(5.1,11.,29.5));
#21668=CARTESIAN_POINT('',(5.2,11.,31.05));
#21669=CARTESIAN_POINT('Origin',(5.2,11.,29.5));
#21670=CARTESIAN_POINT('',(5.,11.,31.25));
#21671=CARTESIAN_POINT('',(5.1,11.,31.15));
#21672=CARTESIAN_POINT('Origin',(5.,11.,29.5));
#21673=CARTESIAN_POINT('Origin',(5.,21.,27.875));
#21674=CARTESIAN_POINT('',(5.,6.3,31.05));
#21675=CARTESIAN_POINT('',(5.,6.3,24.7));
#21676=CARTESIAN_POINT('',(5.,6.3,29.5625));
#21677=CARTESIAN_POINT('',(5.,6.5,31.25));
#21678=CARTESIAN_POINT('',(5.,9.15625000000002,33.90625));
#21679=CARTESIAN_POINT('',(5.,6.,31.25));
#21680=CARTESIAN_POINT('',(5.,17.304,31.25));
#21681=CARTESIAN_POINT('',(5.,6.,31.25));
#21682=CARTESIAN_POINT('',(5.,17.6454213562373,31.1085786437627));
#21683=CARTESIAN_POINT('',(5.,19.5633433515018,30.3141493417505));
#21684=CARTESIAN_POINT('',(5.,20.4,28.354));
#21685=CARTESIAN_POINT('',(5.,17.504,31.25));
#21686=CARTESIAN_POINT('',(5.,20.4,27.154));
#21687=CARTESIAN_POINT('',(5.,20.4,28.354));
#21688=CARTESIAN_POINT('',(5.,21.6,27.154));
#21689=CARTESIAN_POINT('',(5.,20.4,27.154));
#21690=CARTESIAN_POINT('',(5.,21.6,28.354));
#21691=CARTESIAN_POINT('',(5.,21.6,27.154));
#21692=CARTESIAN_POINT('',(5.,24.3545786437627,31.1085786437627));
#21693=CARTESIAN_POINT('',(5.,21.6,28.354));
#21694=CARTESIAN_POINT('',(5.,24.696,31.25));
#21695=CARTESIAN_POINT('',(5.,22.4366566484982,30.3141493417505));
#21696=CARTESIAN_POINT('',(5.,35.5,31.25));
#21697=CARTESIAN_POINT('',(5.,24.496,31.25));
#21698=CARTESIAN_POINT('',(5.,35.7,31.05));
#21699=CARTESIAN_POINT('',(5.,32.84375,33.90625));
#21700=CARTESIAN_POINT('',(5.,35.7,24.7));
#21701=CARTESIAN_POINT('',(5.,35.7,26.1875));
#21702=CARTESIAN_POINT('',(5.,35.5,24.5));
#21703=CARTESIAN_POINT('',(5.,32.84375,21.84375));
#21704=CARTESIAN_POINT('',(5.,6.5,24.5));
#21705=CARTESIAN_POINT('',(5.,36.,24.5));
#21706=CARTESIAN_POINT('',(5.,9.15625000000002,21.84375));
#21707=CARTESIAN_POINT('Origin',(5.,11.,29.5));
#21708=CARTESIAN_POINT('',(12.,11.,31.05));
#21709=CARTESIAN_POINT('',(5.,11.,31.05));
#21710=CARTESIAN_POINT('',(12.,9.45,29.5));
#21711=CARTESIAN_POINT('Origin',(12.,11.,29.5));
#21712=CARTESIAN_POINT('Origin',(12.,11.,29.5));
#21713=CARTESIAN_POINT('Origin',(12.,11.,29.5));
#21714=CARTESIAN_POINT('',(12.9313339594927,11.,29.5));
#21715=CARTESIAN_POINT('',(12.,9.45,29.5));
#21716=CARTESIAN_POINT('Origin',(155.,21.,24.65));
#21717=CARTESIAN_POINT('',(152.45,21.,24.8));
#21718=CARTESIAN_POINT('Origin',(155.,21.,24.8));
#21719=CARTESIAN_POINT('',(152.15,21.,24.5));
#21720=CARTESIAN_POINT('',(152.3,21.,24.65));
#21721=CARTESIAN_POINT('Origin',(155.,21.,24.5));
#21722=CARTESIAN_POINT('Origin',(5.,6.,24.5));
#21723=CARTESIAN_POINT('',(5.,6.5,24.5));
#21724=CARTESIAN_POINT('',(5.,35.5,24.5));
#21725=CARTESIAN_POINT('',(102.15,21.,24.5));
#21726=CARTESIAN_POINT('Origin',(105.,21.,24.5));
#21727=CARTESIAN_POINT('',(52.15,21.,24.5));
#21728=CARTESIAN_POINT('Origin',(55.,21.,24.5));
#21729=CARTESIAN_POINT('Origin',(155.,21.,24.5));
#21730=CARTESIAN_POINT('',(152.45,21.,27.154));
#21731=CARTESIAN_POINT('',(152.45,21.,24.5));
#21732=CARTESIAN_POINT('',(152.521593253721,20.4,27.154));
#21733=CARTESIAN_POINT('Origin',(155.,21.,27.154));
#21734=CARTESIAN_POINT('',(152.521593253721,20.4,28.354));
#21735=CARTESIAN_POINT('',(152.521593253721,20.4,24.5));
#21736=CARTESIAN_POINT('',(152.545690321088,20.308,28.446));
#21737=CARTESIAN_POINT('Origin',(155.,21.,27.754));
#21738=CARTESIAN_POINT('',(157.454309678912,20.308,28.446));
#21739=CARTESIAN_POINT('Origin',(155.,21.,28.446));
#21740=CARTESIAN_POINT('',(157.478406746279,20.4,28.354));
#21741=CARTESIAN_POINT('Origin',(155.,21.,27.754));
#21742=CARTESIAN_POINT('',(157.478406746279,20.4,27.154));
#21743=CARTESIAN_POINT('',(157.478406746279,20.4,24.5));
#21744=CARTESIAN_POINT('',(157.478406746279,21.6,27.154));
#21745=CARTESIAN_POINT('Origin',(155.,21.,27.154));
#21746=CARTESIAN_POINT('',(157.478406746279,21.6,28.354));
#21747=CARTESIAN_POINT('',(157.478406746279,21.6,24.5));
#21748=CARTESIAN_POINT('',(157.454309678912,21.692,28.446));
#21749=CARTESIAN_POINT('Origin',(155.,21.,27.754));
#21750=CARTESIAN_POINT('',(152.545690321088,21.692,28.446));
#21751=CARTESIAN_POINT('Origin',(155.,21.,28.446));
#21752=CARTESIAN_POINT('',(152.521593253721,21.6,28.354));
#21753=CARTESIAN_POINT('Origin',(155.,21.,27.754));
#21754=CARTESIAN_POINT('',(152.521593253721,21.6,27.154));
#21755=CARTESIAN_POINT('',(152.521593253721,21.6,24.5));
#21756=CARTESIAN_POINT('Origin',(155.,21.,27.154));
#21757=CARTESIAN_POINT('Origin',(105.,21.,24.65));
#21758=CARTESIAN_POINT('',(102.45,21.,24.8));
#21759=CARTESIAN_POINT('Origin',(105.,21.,24.8));
#21760=CARTESIAN_POINT('',(102.3,21.,24.65));
#21761=CARTESIAN_POINT('Origin',(105.,21.,24.5));
#21762=CARTESIAN_POINT('',(102.45,21.,27.154));
#21763=CARTESIAN_POINT('',(102.45,21.,24.5));
#21764=CARTESIAN_POINT('',(102.521593253721,20.4,27.154));
#21765=CARTESIAN_POINT('Origin',(105.,21.,27.154));
#21766=CARTESIAN_POINT('',(102.521593253721,20.4,28.354));
#21767=CARTESIAN_POINT('',(102.521593253721,20.4,24.5));
#21768=CARTESIAN_POINT('',(102.545690321088,20.308,28.446));
#21769=CARTESIAN_POINT('Origin',(105.,21.,27.754));
#21770=CARTESIAN_POINT('',(107.454309678912,20.308,28.446));
#21771=CARTESIAN_POINT('Origin',(105.,21.,28.446));
#21772=CARTESIAN_POINT('',(107.478406746279,20.4,28.354));
#21773=CARTESIAN_POINT('Origin',(105.,21.,27.754));
#21774=CARTESIAN_POINT('',(107.478406746279,20.4,27.154));
#21775=CARTESIAN_POINT('',(107.478406746279,20.4,24.5));
#21776=CARTESIAN_POINT('',(107.478406746279,21.6,27.154));
#21777=CARTESIAN_POINT('Origin',(105.,21.,27.154));
#21778=CARTESIAN_POINT('',(107.478406746279,21.6,28.354));
#21779=CARTESIAN_POINT('',(107.478406746279,21.6,24.5));
#21780=CARTESIAN_POINT('',(107.454309678912,21.692,28.446));
#21781=CARTESIAN_POINT('Origin',(105.,21.,27.754));
#21782=CARTESIAN_POINT('',(102.545690321088,21.692,28.446));
#21783=CARTESIAN_POINT('Origin',(105.,21.,28.446));
#21784=CARTESIAN_POINT('',(102.521593253721,21.6,28.354));
#21785=CARTESIAN_POINT('Origin',(105.,21.,27.754));
#21786=CARTESIAN_POINT('',(102.521593253721,21.6,27.154));
#21787=CARTESIAN_POINT('',(102.521593253721,21.6,24.5));
#21788=CARTESIAN_POINT('Origin',(105.,21.,27.154));
#21789=CARTESIAN_POINT('Origin',(55.,21.,24.65));
#21790=CARTESIAN_POINT('',(52.45,21.,24.8));
#21791=CARTESIAN_POINT('Origin',(55.,21.,24.8));
#21792=CARTESIAN_POINT('',(52.3,21.,24.65));
#21793=CARTESIAN_POINT('Origin',(55.,21.,24.5));
#21794=CARTESIAN_POINT('',(52.45,21.,27.154));
#21795=CARTESIAN_POINT('',(52.45,21.,24.5));
#21796=CARTESIAN_POINT('',(52.5215932537213,20.4,27.154));
#21797=CARTESIAN_POINT('Origin',(55.,21.,27.154));
#21798=CARTESIAN_POINT('',(52.5215932537213,20.4,28.354));
#21799=CARTESIAN_POINT('',(52.5215932537213,20.4,24.5));
#21800=CARTESIAN_POINT('',(52.5456903210882,20.308,28.446));
#21801=CARTESIAN_POINT('Origin',(55.,21.,27.754));
#21802=CARTESIAN_POINT('',(57.4543096789118,20.308,28.446));
#21803=CARTESIAN_POINT('Origin',(55.,21.,28.446));
#21804=CARTESIAN_POINT('',(57.4784067462787,20.4,28.354));
#21805=CARTESIAN_POINT('Origin',(55.,21.,27.754));
#21806=CARTESIAN_POINT('',(57.4784067462787,20.4,27.154));
#21807=CARTESIAN_POINT('',(57.4784067462787,20.4,24.5));
#21808=CARTESIAN_POINT('',(57.4784067462787,21.6,27.154));
#21809=CARTESIAN_POINT('Origin',(55.,21.,27.154));
#21810=CARTESIAN_POINT('',(57.4784067462787,21.6,28.354));
#21811=CARTESIAN_POINT('',(57.4784067462787,21.6,24.5));
#21812=CARTESIAN_POINT('',(57.4543096789118,21.692,28.446));
#21813=CARTESIAN_POINT('Origin',(55.,21.,27.754));
#21814=CARTESIAN_POINT('',(52.5456903210882,21.692,28.446));
#21815=CARTESIAN_POINT('Origin',(55.,21.,28.446));
#21816=CARTESIAN_POINT('',(52.5215932537213,21.6,28.354));
#21817=CARTESIAN_POINT('Origin',(55.,21.,27.754));
#21818=CARTESIAN_POINT('',(52.5215932537213,21.6,27.154));
#21819=CARTESIAN_POINT('',(52.5215932537213,21.6,24.5));
#21820=CARTESIAN_POINT('Origin',(55.,21.,27.154));
#21821=CARTESIAN_POINT('Origin',(55.,21.,28.446));
#21822=CARTESIAN_POINT('',(30.,20.308,28.446));
#21823=CARTESIAN_POINT('Origin',(55.,21.,28.446));
#21824=CARTESIAN_POINT('',(30.,21.692,28.446));
#21825=CARTESIAN_POINT('Origin',(105.,21.,28.446));
#21826=CARTESIAN_POINT('',(55.,20.308,28.446));
#21827=CARTESIAN_POINT('Origin',(105.,21.,28.446));
#21828=CARTESIAN_POINT('',(55.,21.692,28.446));
#21829=CARTESIAN_POINT('Origin',(155.,21.,28.446));
#21830=CARTESIAN_POINT('',(80.,20.308,28.446));
#21831=CARTESIAN_POINT('Origin',(155.,21.,28.446));
#21832=CARTESIAN_POINT('',(80.,21.692,28.446));
#21833=CARTESIAN_POINT('Origin',(5.,24.496,31.25));
#21834=CARTESIAN_POINT('',(5.,21.6,28.354));
#21835=CARTESIAN_POINT('',(5.,21.6,28.354));
#21836=CARTESIAN_POINT('',(5.,21.6,28.354));
#21837=CARTESIAN_POINT('',(5.,24.3545786437627,31.1085786437627));
#21838=CARTESIAN_POINT('',(5.,21.6,28.354));
#21839=CARTESIAN_POINT('Origin',(5.,21.6,28.354));
#21840=CARTESIAN_POINT('',(5.,21.6,27.154));
#21841=CARTESIAN_POINT('Origin',(5.,21.6,28.354));
#21842=CARTESIAN_POINT('',(5.,21.6,27.154));
#21843=CARTESIAN_POINT('Origin',(5.,21.6,28.354));
#21844=CARTESIAN_POINT('',(5.,21.6,27.154));
#21845=CARTESIAN_POINT('Origin',(5.,21.6,27.154));
#21846=CARTESIAN_POINT('',(5.,20.4,27.154));
#21847=CARTESIAN_POINT('Origin',(5.,21.6,27.154));
#21848=CARTESIAN_POINT('',(5.,20.4,27.154));
#21849=CARTESIAN_POINT('Origin',(5.,21.6,27.154));
#21850=CARTESIAN_POINT('',(5.,20.4,27.154));
#21851=CARTESIAN_POINT('Origin',(5.,20.4,27.154));
#21852=CARTESIAN_POINT('',(5.,20.4,28.354));
#21853=CARTESIAN_POINT('Origin',(5.,20.4,27.154));
#21854=CARTESIAN_POINT('',(5.,20.4,28.354));
#21855=CARTESIAN_POINT('Origin',(5.,20.4,27.154));
#21856=CARTESIAN_POINT('',(5.,20.4,28.354));
#21857=CARTESIAN_POINT('Origin',(204.85,6.15,29.5625));
#21858=CARTESIAN_POINT('',(204.7,6.,25.));
#21859=CARTESIAN_POINT('',(170.789583333332,-27.9104166666672,58.910416666667));
#21860=CARTESIAN_POINT('',(204.7,6.,30.75));
#21861=CARTESIAN_POINT('',(171.352083333332,-27.3479166666672,-2.59791666666702));
#21862=CARTESIAN_POINT('',(204.7,6.,29.5625));
#21863=CARTESIAN_POINT('Origin',(5.,6.,31.25));
#21864=CARTESIAN_POINT('',(5.3,6.,30.75));
#21865=CARTESIAN_POINT('',(5.,6.,30.75));
#21866=CARTESIAN_POINT('',(5.3,6.,25.));
#21867=CARTESIAN_POINT('',(5.3,6.,29.5625));
#21868=CARTESIAN_POINT('',(5.,6.,25.));
#21869=CARTESIAN_POINT('Origin',(5.,6.25,31.));
#21870=CARTESIAN_POINT('',(5.,6.5,31.25));
#21871=CARTESIAN_POINT('',(5.31458333333333,5.98541666666667,30.7354166666667));
#21872=CARTESIAN_POINT('Origin',(204.85,35.85,26.1875));
#21873=CARTESIAN_POINT('',(204.7,36.,30.75));
#21874=CARTESIAN_POINT('',(170.789583333331,69.9104166666672,-3.16041666666715));
#21875=CARTESIAN_POINT('',(204.7,36.,25.));
#21876=CARTESIAN_POINT('',(171.352083333331,69.3479166666672,58.3479166666672));
#21877=CARTESIAN_POINT('',(204.7,36.,26.1875));
#21878=CARTESIAN_POINT('Origin',(5.,35.75,31.));
#21879=CARTESIAN_POINT('',(5.3,36.,30.75));
#21880=CARTESIAN_POINT('',(5.,36.,30.75));
#21881=CARTESIAN_POINT('',(5.87708333333334,36.5770833333333,30.1729166666667));
#21882=CARTESIAN_POINT('',(5.,35.5,31.25));
#21883=CARTESIAN_POINT('Origin',(5.,36.,24.5));
#21884=CARTESIAN_POINT('',(5.3,36.,25.));
#21885=CARTESIAN_POINT('',(5.,36.,25.));
#21886=CARTESIAN_POINT('',(5.3,36.,26.1875));
#21887=CARTESIAN_POINT('Origin',(5.15,6.15,29.5625));
#21888=CARTESIAN_POINT('',(5.87708333333333,5.42291666666667,25.5770833333333));
#21889=CARTESIAN_POINT('Origin',(5.15,35.85,26.1875));
#21890=CARTESIAN_POINT('',(5.31458333333333,36.0145833333333,25.0145833333333));
#21891=CARTESIAN_POINT('Origin',(5.,24.5252893218813,31.1792893218813));
#21892=CARTESIAN_POINT('',(5.,24.696,31.25));
#21893=CARTESIAN_POINT('Origin',(5.,36.,31.25));
#21894=CARTESIAN_POINT('Origin',(5.,17.4747106781187,31.1792893218813));
#21895=CARTESIAN_POINT('',(5.,17.6454213562373,31.1085786437627));
#21896=CARTESIAN_POINT('',(5.,17.304,31.25));
#21897=CARTESIAN_POINT('Origin',(5.,20.4,28.354));
#21898=CARTESIAN_POINT('',(5.,20.4,28.354));
#21899=CARTESIAN_POINT('Origin',(5.,6.25,24.75));
#21900=CARTESIAN_POINT('Origin',(5.,35.75,24.75));
#21901=CARTESIAN_POINT('Origin',(5.,17.504,31.25));
#21902=CARTESIAN_POINT('Origin',(5.,20.4,27.154));
#21903=CARTESIAN_POINT('',(5.,20.4,27.154));
#21904=CARTESIAN_POINT('Origin',(5.,21.6,27.154));
#21905=CARTESIAN_POINT('',(5.,21.6,27.154));
#21906=CARTESIAN_POINT('Origin',(5.,21.6,28.354));
#81020=UNCERTAINTY_MEASURE_WITH_UNIT(LENGTH_MEASURE(0.01),#81041,
'DISTANCE_ACCURACY_VALUE',
'Maximum model space distance between geometric entities at asserted c
onnectivities');
#81028=UNCERTAINTY_MEASURE_WITH_UNIT(LENGTH_MEASURE(0.01),#81041,
'DISTANCE_ACCURACY_VALUE',
'Maximum model space distance between geometric entities at asserted c
onnectivities');
#81032=(
GEOMETRIC_REPRESENTATION_CONTEXT(3)
GLOBAL_UNCERTAINTY_ASSIGNED_CONTEXT((#81020))
GLOBAL_UNIT_ASSIGNED_CONTEXT((#81041,#81043,#81044))
REPRESENTATION_CONTEXT('','3D')
);
#81040=(
GEOMETRIC_REPRESENTATION_CONTEXT(3)
GLOBAL_UNCERTAINTY_ASSIGNED_CONTEXT((#81028))
GLOBAL_UNIT_ASSIGNED_CONTEXT((#81041,#81043,#81044))
REPRESENTATION_CONTEXT('','3D')
);
#81041=(
LENGTH_UNIT()
NAMED_UNIT(*)
SI_UNIT(.MILLI.,.METRE.)
);
#81043=(
NAMED_UNIT(*)
PLANE_ANGLE_UNIT()
SI_UNIT($,.RADIAN.)
);
#81044=(
NAMED_UNIT(*)
SI_UNIT($,.STERADIAN.)
SOLID_ANGLE_UNIT()
);
#81048=SHAPE_DEFINITION_REPRESENTATION(#81059,#81132);
#81059=PRODUCT_DEFINITION_SHAPE('',$,#81144);
#81132=SHAPE_REPRESENTATION('',(#15614),#81032);
#81140=PRODUCT_DEFINITION_CONTEXT('part definition',#81175,'design');
#81144=PRODUCT_DEFINITION('V-Way Roller Rail Table Side',
'V-Way Roller Rail Table Side',#81155,#81140);
#81155=PRODUCT_DEFINITION_FORMATION('',$,#81180);
#81175=APPLICATION_CONTEXT(
'Core Data for Automotive Mechanical Design Process');
#81176=PRODUCT_CONTEXT('part definition',#81175,'mechanical');
#81180=PRODUCT('V-Way Roller Rail Table Side',
'V-Way Roller Rail Table Side',$,(#81176));
#81191=PRESENTATION_STYLE_ASSIGNMENT((#81202));
#81202=SURFACE_STYLE_USAGE(.BOTH.,#81213);
#81213=SURFACE_SIDE_STYLE('',(#81224));
#81224=SURFACE_STYLE_FILL_AREA(#81235);
#81235=FILL_AREA_STYLE('Opaque(232,234,237)',(#81246));
#81246=FILL_AREA_STYLE_COLOUR('Opaque(232,234,237)',#81257);
#81257=COLOUR_RGB('Opaque(232,234,237)', 0.31764706, 0.68627451, 0.89019608);
ENDSEC;
END-ISO-10303-21;
